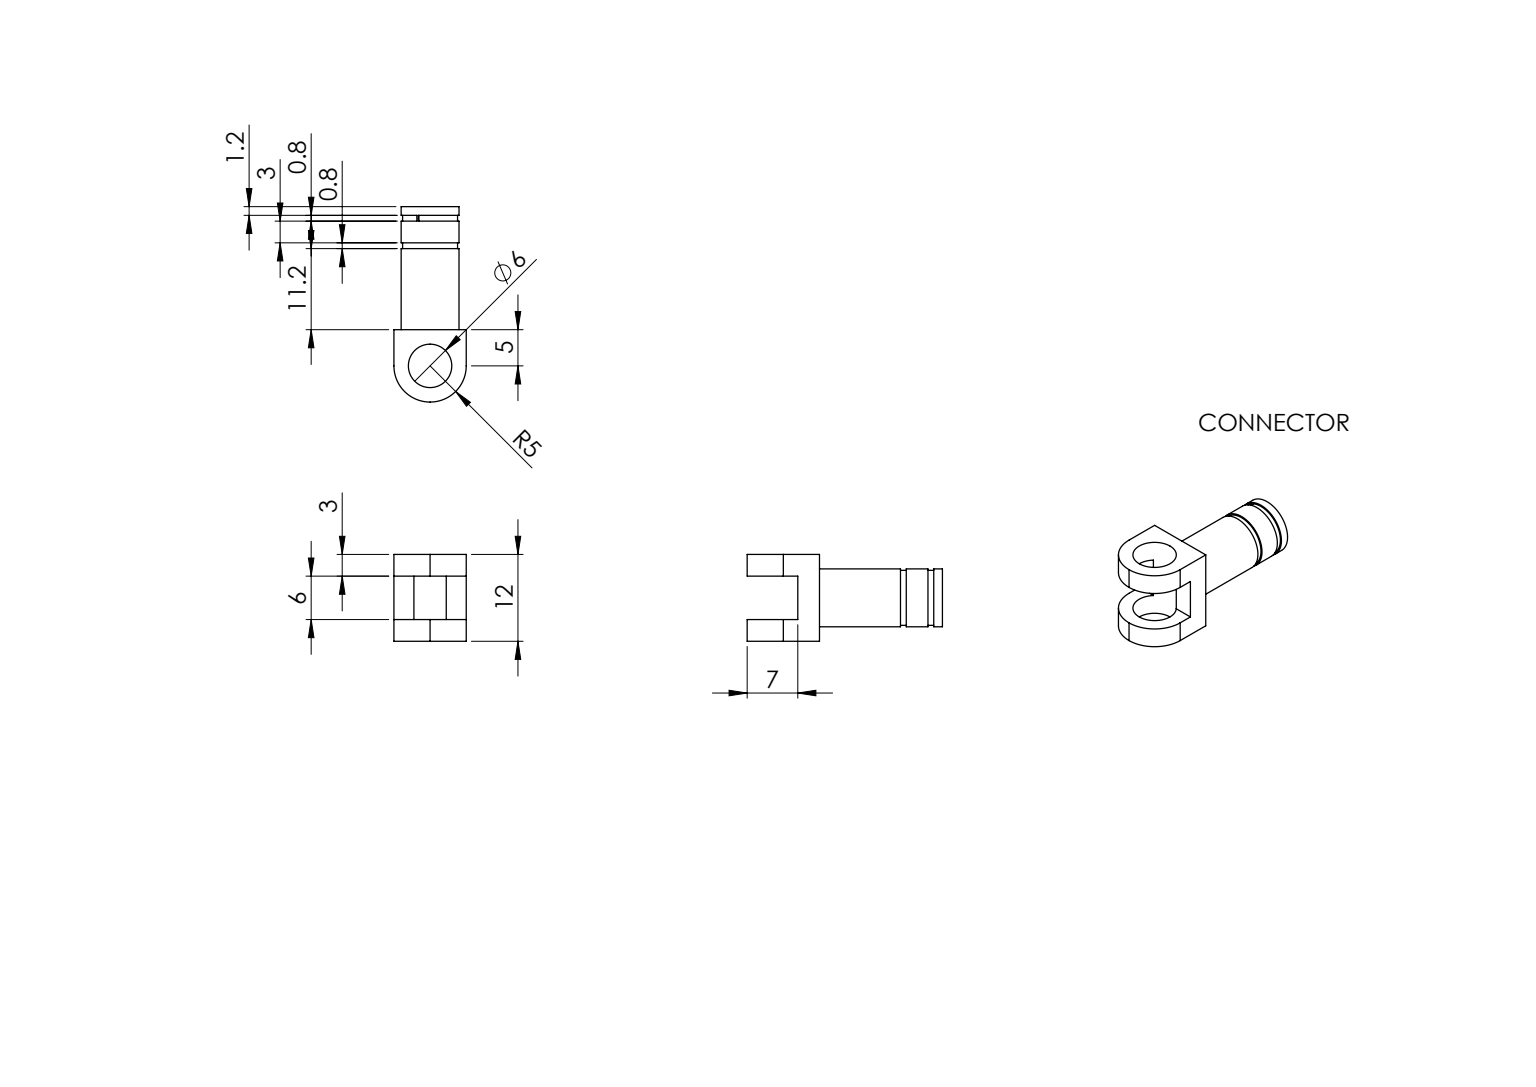
ISO-10303-21;
HEADER;
FILE_DESCRIPTION (('STEP AP214'),
    '1' );
FILE_NAME ('connector.step',
    '2026-10-31T03:41:51',
    ( '' ),
    ( '' ),
    'SwSTEP 2.0',
    'SolidWorks 2026',
    '' );
FILE_SCHEMA (( 'AUTOMOTIVE_DESIGN' ));
ENDSEC;

DATA;
#29=EDGE_CURVE ( 'NONE', #14731, #12050, #4275, .T. ) ;
#49=CARTESIAN_POINT ( 'NONE',  ( -14.40394475573011945, -10.79473832354794460, -3.794707603699265519E-15 ) ) ;
#69=ORIENTED_EDGE ( 'NONE', *, *, #13888, .F. ) ;
#80=EDGE_CURVE ( 'NONE', #14477, #12497, #893, .T. ) ;
#95=CARTESIAN_POINT ( 'NONE',  ( -14.40394475573011945, -2.082238426203170629E-15, 16.99999999999999645 ) ) ;
#102=DIRECTION ( 'NONE',  ( 0.9021244663126475327, 0.4314758942051350465, -1.141265444721583757E-16 ) ) ;
#107=VECTOR ( 'NONE', #15180, 1000.000000000000114 ) ;
#134=VERTEX_POINT ( 'NONE', #3643 ) ;
#139=CIRCLE ( 'NONE', #11189, 3.799999999999999378 ) ;
#140=EDGE_CURVE ( 'NONE', #12264, #4663, #14022, .T. ) ;
#162=CARTESIAN_POINT ( 'NONE',  ( -16.14082873121598993, -7.414910804916202913, -3.000000000000000000 ) ) ;
#189=DIRECTION ( 'NONE',  ( -1.576560579138138762E-17, 1.359337748750801608E-17, -1.000000000000000000 ) ) ;
#194=ORIENTED_EDGE ( 'NONE', *, *, #4990, .T. ) ;
#196=AXIS2_PLACEMENT_3D ( 'NONE', #5704, #8149, #10157 ) ;
#276=ORIENTED_EDGE ( 'NONE', *, *, #3938, .F. ) ;
#298=ORIENTED_EDGE ( 'NONE', *, *, #4470, .F. ) ;
#323=ORIENTED_EDGE ( 'NONE', *, *, #9187, .T. ) ;
#358=ORIENTED_EDGE ( 'NONE', *, *, #7383, .F. ) ;
#377=CARTESIAN_POINT ( 'NONE',  ( -14.40394475573011768, -13.79473832354794993, 16.99999999999999645 ) ) ;
#385=CARTESIAN_POINT ( 'NONE',  ( -16.02604379927987566, -7.138402084508245871, -3.000000000000000444 ) ) ;
#387=AXIS2_PLACEMENT_3D ( 'NONE', #8515, #438, #8738 ) ;
#415=CIRCLE ( 'NONE', #14963, 5.000000000000000888 ) ;
#416=DIRECTION ( 'NONE',  ( 1.576560579138138762E-17, -1.359337748750801608E-17, 1.000000000000000000 ) ) ;
#417=DIRECTION ( 'NONE',  ( 1.000000000000000000, 0.000000000000000000, -0.000000000000000000 ) ) ;
#418=VERTEX_POINT ( 'NONE', #1273 ) ;
#424=DIRECTION ( 'NONE',  ( -1.000000000000000000, 0.000000000000000000, -0.000000000000000000 ) ) ;
#426=CIRCLE ( 'NONE', #5853, 4.999999999999999112 ) ;
#436=DIRECTION ( 'NONE',  ( 1.000000000000000000, 0.000000000000000000, 0.000000000000000000 ) ) ;
#438=DIRECTION ( 'NONE',  ( -0.000000000000000000, -1.000000000000000000, -0.000000000000000000 ) ) ;
#453=EDGE_CURVE ( 'NONE', #2791, #11000, #13669, .T. ) ;
#490=ORIENTED_EDGE ( 'NONE', *, *, #9421, .T. ) ;
#531=CARTESIAN_POINT ( 'NONE',  ( -9.403944755730117677, -13.79473832354794816, 22.00000000000000000 ) ) ;
#532=ADVANCED_FACE ( 'NONE', ( #1053 ), #13021, .T. ) ;
#545=EDGE_CURVE ( 'NONE', #7272, #5145, #11103, .T. ) ;
#547=VECTOR ( 'NONE', #3000, 1000.000000000000000 ) ;
#598=CARTESIAN_POINT ( 'NONE',  ( -17.10144940350364706, -13.74829019802725050, -5.000000000000000000 ) ) ;
#648=DIRECTION ( 'NONE',  ( 0.000000000000000000, 0.000000000000000000, 1.000000000000000000 ) ) ;
#650=ADVANCED_FACE ( 'NONE', ( #7584 ), #3969, .T. ) ;
#653=FACE_OUTER_BOUND ( 'NONE', #7548, .T. ) ;
#667=VECTOR ( 'NONE', #8814, 999.9999999999998863 ) ;
#678=MECHANICAL_DESIGN_GEOMETRIC_PRESENTATION_REPRESENTATION('',(#1413),#6575);
#697=AXIS2_PLACEMENT_3D ( 'NONE', #7574, #6261, #2880 ) ;
#699=DIRECTION ( 'NONE',  ( 0.000000000000000000, 0.000000000000000000, 1.000000000000000000 ) ) ;
#718=DIRECTION ( 'NONE',  ( 1.445602896647338917E-16, -1.000000000000000000, 0.000000000000000000 ) ) ;
#725=ADVANCED_FACE ( 'NONE', ( #9367 ), #12746, .F. ) ;
#735=DIRECTION ( 'NONE',  ( 0.9021244663126475327, 0.4314758942051350465, -1.141265444721583757E-16 ) ) ;
#736=DIRECTION ( 'NONE',  ( -5.782411586589355667E-16, -1.000000000000000000, 0.000000000000000000 ) ) ;
#750=FACE_OUTER_BOUND ( 'NONE', #10103, .T. ) ;
#756=CARTESIAN_POINT ( 'NONE',  ( -15.94493884710238696, -7.321218896460230496, -3.800000000000000266 ) ) ;
#761=VERTEX_POINT ( 'NONE', #8286 ) ;
#782=LINE ( 'NONE', #2247, #5291 ) ;
#784=CARTESIAN_POINT ( 'NONE',  ( -14.40394475573011945, -10.79473832354794460, -3.469446951953614189E-15 ) ) ;
#819=DIRECTION ( 'NONE',  ( 1.000000000000000000, 1.445602896647338424E-16, 0.000000000000000000 ) ) ;
#830=ORIENTED_EDGE ( 'NONE', *, *, #14959, .F. ) ;
#834=ORIENTED_EDGE ( 'NONE', *, *, #13052, .F. ) ;
#851=VERTEX_POINT ( 'NONE', #7377 ) ;
#867=ORIENTED_EDGE ( 'NONE', *, *, #10936, .T. ) ;
#868=DIRECTION ( 'NONE',  ( 0.000000000000000000, 0.000000000000000000, -1.000000000000000000 ) ) ;
#880=ORIENTED_EDGE ( 'NONE', *, *, #7600, .T. ) ;
#893=CIRCLE ( 'NONE', #11692, 4.000000000000000888 ) ;
#923=CARTESIAN_POINT ( 'NONE',  ( -16.14082873121598993, -7.414910804916202913, -3.000000000000000000 ) ) ;
#928=EDGE_LOOP ( 'NONE', ( #1613, #4528 ) ) ;
#968=DIRECTION ( 'NONE',  ( 0.000000000000000000, -1.000000000000000000, 0.000000000000000000 ) ) ;
#972=EDGE_CURVE ( 'NONE', #6697, #12699, #13604, .T. ) ;
#983=ORIENTED_EDGE ( 'NONE', *, *, #14788, .T. ) ;
#988=VERTEX_POINT ( 'NONE', #5302 ) ;
#995=LINE ( 'NONE', #4236, #547 ) ;
#1006=ORIENTED_EDGE ( 'NONE', *, *, #3006, .F. ) ;
#1014=DIRECTION ( 'NONE',  ( -1.445602896647338917E-16, 1.000000000000000000, -0.000000000000000000 ) ) ;
#1022=ORIENTED_EDGE ( 'NONE', *, *, #1967, .T. ) ;
#1025=ORIENTED_EDGE ( 'NONE', *, *, #12744, .F. ) ;
#1036=LINE ( 'NONE', #6952, #3612 ) ;
#1053=FACE_OUTER_BOUND ( 'NONE', #6273, .T. ) ;
#1058=LINE ( 'NONE', #4893, #2111 ) ;
#1069=DIRECTION ( 'NONE',  ( -0.7757024858236036824, 0.6310987668242443727, 2.080818337223229247E-17 ) ) ;
#1076=FILL_AREA_STYLE ('',( #8295 ) ) ;
#1091=VECTOR ( 'NONE', #6616, 1000.000000000000000 ) ;
#1099=CARTESIAN_POINT ( 'NONE',  ( -14.40394475573011235, 8.328953704812679362E-15, 16.99999999999999645 ) ) ;
#1101=EDGE_CURVE ( 'NONE', #4663, #6635, #14169, .T. ) ;
#1107=CYLINDRICAL_SURFACE ( 'NONE', #11751, 4.000000000000000000 ) ;
#1111=DIRECTION ( 'NONE',  ( 1.576560579138138762E-17, -1.359337748750801608E-17, 1.000000000000000000 ) ) ;
#1116=AXIS2_PLACEMENT_3D ( 'NONE', #3202, #7653, #7884 ) ;
#1129=ORIENTED_EDGE ( 'NONE', *, *, #3944, .F. ) ;
#1133=FACE_BOUND ( 'NONE', #9789, .T. ) ;
#1200=CYLINDRICAL_SURFACE ( 'NONE', #10445, 5.000000000000000888 ) ;
#1219=DIRECTION ( 'NONE',  ( 0.000000000000000000, 0.000000000000000000, -1.000000000000000000 ) ) ;
#1227=CIRCLE ( 'NONE', #1977, 4.000000000000000000 ) ;
#1259=EDGE_CURVE ( 'NONE', #9849, #13077, #7974, .T. ) ;
#1270=ORIENTED_EDGE ( 'NONE', *, *, #12382, .F. ) ;
#1271=CARTESIAN_POINT ( 'NONE',  ( -14.40394475573011945, -10.79473832354794460, 0.7999999999999960476 ) ) ;
#1273=CARTESIAN_POINT ( 'NONE',  ( -9.403944755730117677, -13.79473832354794993, 16.99999999999999645 ) ) ;
#1275=VERTEX_POINT ( 'NONE', #1868 ) ;
#1285=EDGE_CURVE ( 'NONE', #14210, #12453, #13387, .T. ) ;
#1288=DIRECTION ( 'NONE',  ( 0.000000000000000000, -1.000000000000000000, 0.000000000000000000 ) ) ;
#1311=PRODUCT_DEFINITION_FORMATION_WITH_SPECIFIED_SOURCE ( 'ANY', '', #13509, .NOT_KNOWN. ) ;
#1349=DIRECTION ( 'NONE',  ( 0.000000000000000000, -1.000000000000000000, 0.000000000000000000 ) ) ;
#1359=CARTESIAN_POINT ( 'NONE',  ( -14.40394475573012301, -13.79473832354794993, 16.99999999999999645 ) ) ;
#1362=AXIS2_PLACEMENT_3D ( 'NONE', #1099, #6945, #14485 ) ;
#1376=AXIS2_PLACEMENT_3D ( 'NONE', #7353, #6187, #9640 ) ;
#1395=VECTOR ( 'NONE', #11283, 1000.000000000000000 ) ;
#1399=EDGE_CURVE ( 'NONE', #6697, #5334, #782, .T. ) ;
#1413=STYLED_ITEM('',(#15258),#13940);
#1414=ORIENTED_EDGE ( 'NONE', *, *, #6168, .F. ) ;
#1435=CARTESIAN_POINT ( 'NONE',  ( -19.40394475573011590, -4.794738323547945491, 12.00000000000000000 ) ) ;
#1441=AXIS2_PLACEMENT_3D ( 'NONE', #14034, #11793, #15127 ) ;
#1456=FACE_OUTER_BOUND ( 'NONE', #5574, .T. ) ;
#1485=VERTEX_POINT ( 'NONE', #10550 ) ;
#1490=LINE ( 'NONE', #1557, #4783 ) ;
#1491=ORIENTED_EDGE ( 'NONE', *, *, #1285, .T. ) ;
#1497=ORIENTED_EDGE ( 'NONE', *, *, #6234, .F. ) ;
#1529=LINE ( 'NONE', #7454, #4580 ) ;
#1543=EDGE_CURVE ( 'NONE', #8254, #761, #13055, .T. ) ;
#1557=CARTESIAN_POINT ( 'NONE',  ( -14.40394475573012301, -4.794738323547945491, 19.99999999999999645 ) ) ;
#1558=EDGE_CURVE ( 'NONE', #2099, #14023, #9734, .T. ) ;
#1587=AXIS2_PLACEMENT_3D ( 'NONE', #4100, #5260, #8780 ) ;
#1598=( GEOMETRIC_REPRESENTATION_CONTEXT ( 3 ) GLOBAL_UNCERTAINTY_ASSIGNED_CONTEXT ( ( #5190 ) ) GLOBAL_UNIT_ASSIGNED_CONTEXT ( ( #5513, #14057, #4970 ) ) REPRESENTATION_CONTEXT ( 'NONE', 'WORKASPACE' ) );
#1611=DIRECTION ( 'NONE',  ( -0.000000000000000000, -1.000000000000000000, -0.000000000000000000 ) ) ;
#1613=ORIENTED_EDGE ( 'NONE', *, *, #13229, .T. ) ;
#1619=CIRCLE ( 'NONE', #1856, 3.799999999999998934 ) ;
#1621=PLANE ( 'NONE',  #11146 ) ;
#1629=ORIENTED_EDGE ( 'NONE', *, *, #7674, .T. ) ;
#1644=VECTOR ( 'NONE', #11061, 1000.000000000000000 ) ;
#1664=DIRECTION ( 'NONE',  ( 0.7573544145849105957, -0.6530040510661073716, -2.081668171172162967E-17 ) ) ;
#1722=ADVANCED_FACE ( 'NONE', ( #3853 ), #11070, .F. ) ;
#1760=CARTESIAN_POINT ( 'NONE',  ( -9.403944755730117677, -16.79473832354794993, 22.00000000000000000 ) ) ;
#1809=ADVANCED_FACE ( 'NONE', ( #3165 ), #13829, .T. ) ;
#1813=VERTEX_POINT ( 'NONE', #7767 ) ;
#1817=CIRCLE ( 'NONE', #8933, 4.000000000000000000 ) ;
#1834=CARTESIAN_POINT ( 'NONE',  ( -16.64001273322991281, -7.794738323547949932, 14.99999999999999822 ) ) ;
#1846=EDGE_CURVE ( 'NONE', #3700, #6635, #6624, .T. ) ;
#1856=AXIS2_PLACEMENT_3D ( 'NONE', #6396, #6233, #3013 ) ;
#1862=CARTESIAN_POINT ( 'NONE',  ( -14.40394475573011945, -10.79473832354794460, 12.00000000000000000 ) ) ;
#1868=CARTESIAN_POINT ( 'NONE',  ( -18.40394475573011945, -10.79473832354794460, -3.406384528788088688E-15 ) ) ;
#1873=EDGE_CURVE ( 'NONE', #3107, #988, #9246, .T. ) ;
#1882=ADVANCED_FACE ( 'NONE', ( #4312 ), #10075, .F. ) ;
#1885=VERTEX_POINT ( 'NONE', #10148 ) ;
#1887=DIRECTION ( 'NONE',  ( -0.000000000000000000, -0.000000000000000000, -1.000000000000000000 ) ) ;
#1909=ORIENTED_EDGE ( 'NONE', *, *, #13404, .F. ) ;
#1926=FACE_OUTER_BOUND ( 'NONE', #4356, .T. ) ;
#1945=AXIS2_PLACEMENT_3D ( 'NONE', #10428, #416, #1664 ) ;
#1954=VECTOR ( 'NONE', #13085, 999.9999999999998863 ) ;
#1967=EDGE_CURVE ( 'NONE', #8601, #9577, #139, .T. ) ;
#1973=DIRECTION ( 'NONE',  ( 0.9021244663126475327, 0.4314758942051350465, -1.141265444721583757E-16 ) ) ;
#1975=DIRECTION ( 'NONE',  ( -5.480158469902919838E-17, -1.051478716308701618E-16, -1.000000000000000000 ) ) ;
#1977=AXIS2_PLACEMENT_3D ( 'NONE', #2826, #14447, #13201 ) ;
#1982=LINE ( 'NONE', #11413, #7043 ) ;
#2027=ORIENTED_EDGE ( 'NONE', *, *, #9884, .T. ) ;
#2040=ORIENTED_EDGE ( 'NONE', *, *, #3738, .F. ) ;
#2084=AXIS2_PLACEMENT_3D ( 'NONE', #4593, #2122, #6813 ) ;
#2092=AXIS2_PLACEMENT_3D ( 'NONE', #9331, #4571, #9393 ) ;
#2099=VERTEX_POINT ( 'NONE', #7603 ) ;
#2111=VECTOR ( 'NONE', #11579, 1000.000000000000000 ) ;
#2113=ADVANCED_FACE ( 'NONE', ( #6290 ), #14525, .F. ) ;
#2118=DIRECTION ( 'NONE',  ( 0.9021244663126475327, 0.4314758942051350465, -1.141265444721583757E-16 ) ) ;
#2122=DIRECTION ( 'NONE',  ( -1.576560579138138762E-17, 1.359337748750801608E-17, -1.000000000000000000 ) ) ;
#2152=DIRECTION ( 'NONE',  ( -5.480158469902919838E-17, -1.051478716308701618E-16, -1.000000000000000000 ) ) ;
#2167=ORIENTED_EDGE ( 'NONE', *, *, #3111, .F. ) ;
#2220=VERTEX_POINT ( 'NONE', #12514 ) ;
#2233=DIRECTION ( 'NONE',  ( 1.445602896647338917E-16, -1.000000000000000000, 0.000000000000000000 ) ) ;
#2243=CARTESIAN_POINT ( 'NONE',  ( -19.40394475573012301, -7.794738323547950820, 16.99999999999999645 ) ) ;
#2247=CARTESIAN_POINT ( 'NONE',  ( -14.40394475573011945, -4.794738323547946379, 22.00000000000000000 ) ) ;
#2252=CARTESIAN_POINT ( 'NONE',  ( -14.40394475573011945, -10.79473832354794460, -5.000000000000000000 ) ) ;
#2268=ORIENTED_EDGE ( 'NONE', *, *, #5962, .F. ) ;
#2275=DIRECTION ( 'NONE',  ( -1.445602896647338917E-16, 1.000000000000000000, -0.000000000000000000 ) ) ;
#2284=CARTESIAN_POINT ( 'NONE',  ( -14.40394475573012301, -16.79473832354794993, 16.99999999999999645 ) ) ;
#2297=EDGE_LOOP ( 'NONE', ( #4906, #13957, #12309, #12977, #13907, #1270, #11727, #7776 ) ) ;
#2302=SURFACE_SIDE_STYLE ('',( #12976 ) ) ;
#2332=DIRECTION ( 'NONE',  ( -0.000000000000000000, -1.000000000000000000, -0.000000000000000000 ) ) ;
#2333=FACE_OUTER_BOUND ( 'NONE', #13646, .T. ) ;
#2336=CYLINDRICAL_SURFACE ( 'NONE', #11386, 4.000000000000000000 ) ;
#2421=CARTESIAN_POINT ( 'NONE',  ( -10.40394475573011945, -10.79473832354794460, -3.532509375119139690E-15 ) ) ;
#2456=DIRECTION ( 'NONE',  ( -0.000000000000000000, 1.000000000000000000, -0.000000000000000000 ) ) ;
#2475=VERTEX_POINT ( 'NONE', #9728 ) ;
#2491=CARTESIAN_POINT ( 'NONE',  ( -16.23224367729419271, -7.237025146040848789, -5.000000000000000000 ) ) ;
#2543=DIRECTION ( 'NONE',  ( 0.6743761619433820131, 0.7383879686198261405, -5.947623346206184252E-19 ) ) ;
#2546=DIRECTION ( 'NONE',  ( 5.782411586589355667E-16, 1.000000000000000000, 0.000000000000000000 ) ) ;
#2558=LINE ( 'NONE', #6539, #4527 ) ;
#2571=CIRCLE ( 'NONE', #3066, 4.000000000000000000 ) ;
#2585=ORIENTED_EDGE ( 'NONE', *, *, #5962, .T. ) ;
#2608=AXIS2_PLACEMENT_3D ( 'NONE', #2988, #7751, #8897 ) ;
#2620=ADVANCED_FACE ( 'NONE', ( #14802 ), #7885, .T. ) ;
#2638=VECTOR ( 'NONE', #13736, 1000.000000000000000 ) ;
#2659=VECTOR ( 'NONE', #12856, 1000.000000000000000 ) ;
#2670=FACE_OUTER_BOUND ( 'NONE', #10290, .T. ) ;
#2676=VECTOR ( 'NONE', #1887, 1000.000000000000000 ) ;
#2684=ORIENTED_EDGE ( 'NONE', *, *, #10788, .F. ) ;
#2687=ORIENTED_EDGE ( 'NONE', *, *, #6331, .F. ) ;
#2688=CARTESIAN_POINT ( 'NONE',  ( -19.40394475573012301, -16.79473832354794993, 12.00000000000000000 ) ) ;
#2692=ORIENTED_EDGE ( 'NONE', *, *, #13890, .T. ) ;
#2703=ADVANCED_FACE ( 'NONE', ( #653 ), #12631, .T. ) ;
#2708=EDGE_CURVE ( 'NONE', #5145, #10081, #5437, .T. ) ;
#2717=PLANE ( 'NONE',  #13142 ) ;
#2719=CARTESIAN_POINT ( 'NONE',  ( -9.403944755730119454, -4.794738323547945491, 14.99999999999999822 ) ) ;
#2791=VERTEX_POINT ( 'NONE', #6950 ) ;
#2796=ORIENTED_EDGE ( 'NONE', *, *, #8740, .T. ) ;
#2797=CARTESIAN_POINT ( 'NONE',  ( -10.40394475573011945, -10.79473832354794460, 12.00000000000000000 ) ) ;
#2804=LINE ( 'NONE', #14653, #2676 ) ;
#2809=DIRECTION ( 'NONE',  ( -1.000000000000000000, -0.000000000000000000, -0.000000000000000000 ) ) ;
#2826=CARTESIAN_POINT ( 'NONE',  ( -14.40394475573011945, -10.79473832354794460, -3.469446951953614189E-15 ) ) ;
#2843=DIRECTION ( 'NONE',  ( 0.000000000000000000, -1.000000000000000000, 0.000000000000000000 ) ) ;
#2880=DIRECTION ( 'NONE',  ( 0.6743761619433820131, 0.7383879686198261405, -5.947623346206184252E-19 ) ) ;
#2881=CIRCLE ( 'NONE', #12200, 4.000000000000000000 ) ;
#2886=DIRECTION ( 'NONE',  ( 1.576560579138138762E-17, -1.359337748750801608E-17, 1.000000000000000000 ) ) ;
#2891=AXIS2_PLACEMENT_3D ( 'NONE', #12339, #14440, #424 ) ;
#2899=ORIENTED_EDGE ( 'NONE', *, *, #5713, .T. ) ;
#2902=DIRECTION ( 'NONE',  ( -0.000000000000000000, -1.000000000000000000, -0.000000000000000000 ) ) ;
#2929=EDGE_CURVE ( 'NONE', #134, #2475, #2558, .T. ) ;
#2937=EDGE_LOOP ( 'NONE', ( #11951, #5390, #3768, #9077, #3420, #14158, #8321, #10483 ) ) ;
#2947=AXIS2_PLACEMENT_3D ( 'NONE', #12814, #1288, #9302 ) ;
#2966=CARTESIAN_POINT ( 'NONE',  ( -11.52599798030746037, -13.27615371759915242, 0.7999999999999959366 ) ) ;
#2971=VERTEX_POINT ( 'NONE', #6460 ) ;
#2974=CARTESIAN_POINT ( 'NONE',  ( -16.14082873121598993, -7.414910804916202913, -3.000000000000000000 ) ) ;
#2976=SHAPE_DEFINITION_REPRESENTATION ( #5300, #10044 ) ;
#2988=CARTESIAN_POINT ( 'NONE',  ( -19.40394475573012301, -7.794738323547950820, 14.99999999999999822 ) ) ;
#2996=EDGE_CURVE ( 'NONE', #4663, #418, #6389, .T. ) ;
#3000=DIRECTION ( 'NONE',  ( 0.000000000000000000, 0.000000000000000000, -1.000000000000000000 ) ) ;
#3006=EDGE_CURVE ( 'NONE', #13883, #14059, #13088, .T. ) ;
#3013=DIRECTION ( 'NONE',  ( 0.7573544145849105957, -0.6530040510661073716, -2.853163611803960010E-17 ) ) ;
#3020=CIRCLE ( 'NONE', #10140, 3.000000000000000888 ) ;
#3035=DIRECTION ( 'NONE',  ( 0.000000000000000000, 1.000000000000000000, -1.084202172485504187E-16 ) ) ;
#3059=ORIENTED_EDGE ( 'NONE', *, *, #14913, .F. ) ;
#3066=AXIS2_PLACEMENT_3D ( 'NONE', #14467, #3933, #12294 ) ;
#3068=CARTESIAN_POINT ( 'NONE',  ( -19.40394475573012301, -7.794738323547950820, 14.99999999999999822 ) ) ;
#3077=VECTOR ( 'NONE', #6509, 999.9999999999998863 ) ;
#3106=VECTOR ( 'NONE', #10371, 1000.000000000000000 ) ;
#3107=VERTEX_POINT ( 'NONE', #923 ) ;
#3111=EDGE_CURVE ( 'NONE', #10457, #12375, #5519, .T. ) ;
#3120=DIRECTION ( 'NONE',  ( -5.480158469902919838E-17, -1.051478716308701618E-16, -1.000000000000000000 ) ) ;
#3141=DIRECTION ( 'NONE',  ( 0.000000000000000000, 0.000000000000000000, 1.000000000000000000 ) ) ;
#3156=CARTESIAN_POINT ( 'NONE',  ( -14.40394475573011945, -4.794738323547946379, 22.00000000000000000 ) ) ;
#3165=FACE_OUTER_BOUND ( 'NONE', #12101, .T. ) ;
#3167=CIRCLE ( 'NONE', #1441, 4.000000000000000888 ) ;
#3173=ORIENTED_EDGE ( 'NONE', *, *, #2929, .T. ) ;
#3195=EDGE_CURVE ( 'NONE', #12453, #8792, #5770, .T. ) ;
#3196=AXIS2_PLACEMENT_3D ( 'NONE', #13510, #7965, #11195 ) ;
#3202=CARTESIAN_POINT ( 'NONE',  ( -14.40394475573011945, -10.79473832354794460, -3.799999999999999822 ) ) ;
#3210=EDGE_LOOP ( 'NONE', ( #8081, #14742, #11925, #14374, #11488 ) ) ;
#3211=CARTESIAN_POINT ( 'NONE',  ( -18.40394475573011945, -10.79473832354794460, 12.00000000000000000 ) ) ;
#3213=CARTESIAN_POINT ( 'NONE',  ( -14.40394475573012301, -16.79473832354794993, 16.99999999999999645 ) ) ;
#3223=FACE_OUTER_BOUND ( 'NONE', #6680, .T. ) ;
#3226=ORIENTED_EDGE ( 'NONE', *, *, #11081, .T. ) ;
#3252=ADVANCED_FACE ( 'NONE', ( #6143 ), #11667, .F. ) ;
#3262=ORIENTED_EDGE ( 'NONE', *, *, #8026, .T. ) ;
#3264=CARTESIAN_POINT ( 'NONE',  ( -14.40394475573012301, -4.794738323547945491, 19.99999999999999645 ) ) ;
#3275=ADVANCED_FACE ( 'NONE', ( #1456 ), #9668, .T. ) ;
#3318=CARTESIAN_POINT ( 'NONE',  ( -14.40394475573011235, 8.328953704812679362E-15, 16.99999999999999645 ) ) ;
#3336=CARTESIAN_POINT ( 'NONE',  ( -14.40394475573011945, -10.79473832354794283, -3.000000000000000000 ) ) ;
#3372=EDGE_LOOP ( 'NONE', ( #4026, #6931, #12680, #15039 ) ) ;
#3379=CARTESIAN_POINT ( 'NONE',  ( -9.403944755730117677, -7.794738323547949044, 16.99999999999999645 ) ) ;
#3387=CARTESIAN_POINT ( 'NONE',  ( -14.40394475573012301, -7.794738323547949932, 16.99999999999999645 ) ) ;
#3417=EDGE_CURVE ( 'NONE', #9424, #14731, #8596, .T. ) ;
#3420=ORIENTED_EDGE ( 'NONE', *, *, #10811, .F. ) ;
#3437=CIRCLE ( 'NONE', #2947, 3.000000000000000888 ) ;
#3457=DIRECTION ( 'NONE',  ( -0.000000000000000000, 1.000000000000000000, -0.000000000000000000 ) ) ;
#3476=ORIENTED_EDGE ( 'NONE', *, *, #545, .F. ) ;
#3479=VERTEX_POINT ( 'NONE', #756 ) ;
#3482=DIRECTION ( 'NONE',  ( 0.000000000000000000, 0.000000000000000000, 1.000000000000000000 ) ) ;
#3489=EDGE_LOOP ( 'NONE', ( #9090, #13919, #13117, #10177, #298, #867, #4996, #9921 ) ) ;
#3496=LINE ( 'NONE', #5822, #6007 ) ;
#3514=CARTESIAN_POINT ( 'NONE',  ( -19.40394475573012301, -7.794738323547950820, 16.99999999999999645 ) ) ;
#3517=EDGE_CURVE ( 'NONE', #13077, #14623, #6897, .T. ) ;
#3520=MECHANICAL_DESIGN_GEOMETRIC_PRESENTATION_REPRESENTATION('',(#8429),#1598);
#3539=EDGE_CURVE ( 'NONE', #6635, #10618, #5457, .T. ) ;
#3563=ADVANCED_FACE ( 'NONE', ( #1133, #7196 ), #3582, .F. ) ;
#3564=CARTESIAN_POINT ( 'NONE',  ( -19.40394475573012301, -13.79473832354794993, 14.99999999999999822 ) ) ;
#3567=AXIS2_PLACEMENT_3D ( 'NONE', #9388, #11911, #2546 ) ;
#3569=CARTESIAN_POINT ( 'NONE',  ( -17.83201772771817772, -12.43434672152745613, -3.799999999999999378 ) ) ;
#3578=ORIENTED_EDGE ( 'NONE', *, *, #9884, .F. ) ;
#3582=PLANE ( 'NONE',  #14156 ) ;
#3597=ORIENTED_EDGE ( 'NONE', *, *, #7049, .F. ) ;
#3612=VECTOR ( 'NONE', #4581, 1000.000000000000000 ) ;
#3614=DIRECTION ( 'NONE',  ( 0.9021244663126474217, 0.4314758942051349910, -9.480662228539549174E-17 ) ) ;
#3626=AXIS2_PLACEMENT_3D ( 'NONE', #13734, #12507, #4279 ) ;
#3641=AXIS2_PLACEMENT_3D ( 'NONE', #11261, #6655, #735 ) ;
#3643=CARTESIAN_POINT ( 'NONE',  ( -19.40394475573012301, -13.79473832354794993, 14.99999999999999822 ) ) ;
#3654=DIRECTION ( 'NONE',  ( 0.000000000000000000, 0.000000000000000000, 1.000000000000000000 ) ) ;
#3688=DIRECTION ( 'NONE',  ( -5.480158469902917989E-17, -1.051478716308701742E-16, -1.000000000000000000 ) ) ;
#3700=VERTEX_POINT ( 'NONE', #4129 ) ;
#3710=DIRECTION ( 'NONE',  ( 1.000000000000000000, 0.000000000000000000, 0.000000000000000000 ) ) ;
#3732=ADVANCED_FACE ( 'NONE', ( #2670 ), #8493, .T. ) ;
#3735=VERTEX_POINT ( 'NONE', #2966 ) ;
#3738=EDGE_CURVE ( 'NONE', #1885, #13883, #4978, .T. ) ;
#3768=ORIENTED_EDGE ( 'NONE', *, *, #3111, .T. ) ;
#3779=ORIENTED_EDGE ( 'NONE', *, *, #4004, .T. ) ;
#3793=CARTESIAN_POINT ( 'NONE',  ( -16.23224367729419271, -7.237025146040845236, -3.000000000000000444 ) ) ;
#3829=CARTESIAN_POINT ( 'NONE',  ( -16.92833982302709828, -13.89754826684236200, -3.471826001292096363E-15 ) ) ;
#3832=DIRECTION ( 'NONE',  ( -5.480158469902919838E-17, -1.051478716308701618E-16, -1.000000000000000000 ) ) ;
#3849=AXIS2_PLACEMENT_3D ( 'NONE', #4003, #8674, #5099 ) ;
#3853=FACE_OUTER_BOUND ( 'NONE', #6301, .T. ) ;
#3866=AXIS2_PLACEMENT_3D ( 'NONE', #7153, #14378, #102 ) ;
#3904=VECTOR ( 'NONE', #15045, 1000.000000000000000 ) ;
#3918=AXIS2_PLACEMENT_3D ( 'NONE', #377, #8672, #10912 ) ;
#3933=DIRECTION ( 'NONE',  ( 1.576560579138138762E-17, -1.359337748750801608E-17, 1.000000000000000000 ) ) ;
#3938=EDGE_CURVE ( 'NONE', #14803, #9849, #1036, .T. ) ;
#3941=EDGE_LOOP ( 'NONE', ( #7656, #7213, #4630, #8940, #7923, #14872, #14071, #4635 ) ) ;
#3944=EDGE_CURVE ( 'NONE', #3945, #1275, #2881, .T. ) ;
#3945=VERTEX_POINT ( 'NONE', #2421 ) ;
#3969=CYLINDRICAL_SURFACE ( 'NONE', #12493, 3.799999999999998934 ) ;
#3973=ORIENTED_EDGE ( 'NONE', *, *, #13888, .T. ) ;
#4003=CARTESIAN_POINT ( 'NONE',  ( -16.14082873121598993, -7.414910804916202913, -3.000000000000000000 ) ) ;
#4004=EDGE_CURVE ( 'NONE', #851, #12497, #9560, .T. ) ;
#4019=EDGE_CURVE ( 'NONE', #3700, #10457, #3020, .T. ) ;
#4026=ORIENTED_EDGE ( 'NONE', *, *, #8740, .F. ) ;
#4046=DIRECTION ( 'NONE',  ( 0.000000000000000000, 0.000000000000000000, 1.000000000000000000 ) ) ;
#4049=CIRCLE ( 'NONE', #7971, 3.000000000000000888 ) ;
#4054=CYLINDRICAL_SURFACE ( 'NONE', #6084, 3.000000000000000888 ) ;
#4067=EDGE_LOOP ( 'NONE', ( #13062, #11992, #7774, #1629 ) ) ;
#4073=VECTOR ( 'NONE', #7837, 1000.000000000000000 ) ;
#4078=DIRECTION ( 'NONE',  ( -1.576560579138138762E-17, 1.359337748750801608E-17, -1.000000000000000000 ) ) ;
#4094=UNCERTAINTY_MEASURE_WITH_UNIT (LENGTH_MEASURE( 1.000000000000000082E-05 ), #10539, 'distance_accuracy_value', 'NONE');
#4100=CARTESIAN_POINT ( 'NONE',  ( -14.40394475573011945, -10.79473832354794460, -3.794707603699265519E-15 ) ) ;
#4129=CARTESIAN_POINT ( 'NONE',  ( -12.16787677823033142, -7.794738323547949932, 14.99999999999999822 ) ) ;
#4142=DIRECTION ( 'NONE',  ( 1.000000000000000000, 0.000000000000000000, 0.000000000000000000 ) ) ;
#4144=DIRECTION ( 'NONE',  ( 1.576560579138138762E-17, -1.359337748750801608E-17, 1.000000000000000000 ) ) ;
#4184=DIRECTION ( 'NONE',  ( 1.576560579138138762E-17, -1.359337748750801608E-17, 1.000000000000000000 ) ) ;
#4200=DIRECTION ( 'NONE',  ( -0.000000000000000000, -1.000000000000000000, -0.000000000000000000 ) ) ;
#4201=DIRECTION ( 'NONE',  ( 0.000000000000000000, 0.000000000000000000, 1.000000000000000000 ) ) ;
#4210=LINE ( 'NONE', #7736, #4612 ) ;
#4217=EDGE_CURVE ( 'NONE', #5125, #134, #5351, .T. ) ;
#4236=CARTESIAN_POINT ( 'NONE',  ( -19.40394475573012301, -13.79473832354794993, 16.99999999999999645 ) ) ;
#4238=CARTESIAN_POINT ( 'NONE',  ( -15.94493884710238696, -7.321218896460230496, -3.000000000000000000 ) ) ;
#4255=DIRECTION ( 'NONE',  ( 1.000000000000000000, 1.734723475976807341E-16, 2.081668171172168908E-15 ) ) ;
#4275=LINE ( 'NONE', #14736, #10383 ) ;
#4279=DIRECTION ( 'NONE',  ( 0.000000000000000000, 1.000000000000000000, -1.084202172485504187E-16 ) ) ;
#4312=FACE_OUTER_BOUND ( 'NONE', #12524, .T. ) ;
#4338=CARTESIAN_POINT ( 'NONE',  ( -10.97587178374205941, -9.155129925568431304, -3.000000000000000444 ) ) ;
#4356=EDGE_LOOP ( 'NONE', ( #14181, #9341, #11503, #9338, #8459 ) ) ;
#4394=DIRECTION ( 'NONE',  ( 0.9021244663126474217, 0.4314758942051349910, -9.480662228539549174E-17 ) ) ;
#4408=VECTOR ( 'NONE', #2809, 1000.000000000000000 ) ;
#4409=VECTOR ( 'NONE', #11012, 1000.000000000000000 ) ;
#4470=EDGE_CURVE ( 'NONE', #10878, #134, #995, .T. ) ;
#4479=LINE ( 'NONE', #9160, #6865 ) ;
#4498=CYLINDRICAL_SURFACE ( 'NONE', #9794, 3.799999999999999378 ) ;
#4514=CARTESIAN_POINT ( 'NONE',  ( -19.40394475573011590, -4.794738323547945491, 16.99999999999999645 ) ) ;
#4523=CARTESIAN_POINT ( 'NONE',  ( -12.16787677823033142, -13.79473832354794993, 14.99999999999999822 ) ) ;
#4524=CARTESIAN_POINT ( 'NONE',  ( -16.92833982302709828, -13.89754826684236200, 0.7999999999999960476 ) ) ;
#4527=VECTOR ( 'NONE', #11071, 1000.000000000000000 ) ;
#4528=ORIENTED_EDGE ( 'NONE', *, *, #12744, .T. ) ;
#4550=CARTESIAN_POINT ( 'NONE',  ( -14.40394475573011945, -10.79473832354794460, -5.000000000000000000 ) ) ;
#4551=CIRCLE ( 'NONE', #2084, 3.799999999999998934 ) ;
#4557=DIRECTION ( 'NONE',  ( -5.480158469902919838E-17, -1.051478716308701618E-16, -1.000000000000000000 ) ) ;
#4571=DIRECTION ( 'NONE',  ( 1.576560579138138762E-17, -1.359337748750801762E-17, 1.000000000000000000 ) ) ;
#4580=VECTOR ( 'NONE', #1611, 1000.000000000000000 ) ;
#4581=DIRECTION ( 'NONE',  ( 0.6743761619433820131, 0.7383879686198261405, -5.947623346206184252E-19 ) ) ;
#4584=EDGE_LOOP ( 'NONE', ( #9033, #11682, #11208, #14116, #11428, #13711, #10453, #2167 ) ) ;
#4593=CARTESIAN_POINT ( 'NONE',  ( -14.40394475573011945, -10.79473832354794460, 0.7999999999999960476 ) ) ;
#4612=VECTOR ( 'NONE', #13648, 1000.000000000000000 ) ;
#4630=ORIENTED_EDGE ( 'NONE', *, *, #13966, .T. ) ;
#4635=ORIENTED_EDGE ( 'NONE', *, *, #4019, .T. ) ;
#4650=CARTESIAN_POINT ( 'NONE',  ( -10.40394475573011945, -10.79473832354794460, 0.7999999999999959366 ) ) ;
#4655=PLANE ( 'NONE',  #2092 ) ;
#4663=VERTEX_POINT ( 'NONE', #10889 ) ;
#4757=LINE ( 'NONE', #4920, #9449 ) ;
#4781=CARTESIAN_POINT ( 'NONE',  ( -14.40394475573011945, -10.79473832354794283, -3.799999999999999822 ) ) ;
#4783=VECTOR ( 'NONE', #7484, 1000.000000000000000 ) ;
#4815=CARTESIAN_POINT ( 'NONE',  ( -17.83201772771817772, -12.43434672152745613, -2.999999999999999556 ) ) ;
#4822=EDGE_LOOP ( 'NONE', ( #11425, #3597, #7785, #3476 ) ) ;
#4825=DIRECTION ( 'NONE',  ( 0.000000000000000000, 0.000000000000000000, -1.000000000000000000 ) ) ;
#4836=DIRECTION ( 'NONE',  ( 0.000000000000000000, 1.000000000000000000, 0.000000000000000000 ) ) ;
#4893=CARTESIAN_POINT ( 'NONE',  ( -9.403944755730119454, -4.794738323547945491, 22.00000000000000000 ) ) ;
#4902=AXIS2_PLACEMENT_3D ( 'NONE', #10449, #1069, #14051 ) ;
#4906=ORIENTED_EDGE ( 'NONE', *, *, #1101, .F. ) ;
#4912=ADVANCED_BREP_SHAPE_REPRESENTATION ( '', ( #13940, #1376 ), #9175 ) ;
#4913=CIRCLE ( 'NONE', #3918, 4.999999999999999112 ) ;
#4920=CARTESIAN_POINT ( 'NONE',  ( -12.16787677823033142, -4.794738323547945491, 14.99999999999999822 ) ) ;
#4927=LINE ( 'NONE', #9596, #14190 ) ;
#4932=PRESENTATION_STYLE_ASSIGNMENT (( #5988 ) ) ;
#4944=ORIENTED_EDGE ( 'NONE', *, *, #10881, .F. ) ;
#4949=ORIENTED_EDGE ( 'NONE', *, *, #1846, .F. ) ;
#4955=VECTOR ( 'NONE', #718, 1000.000000000000000 ) ;
#4970=( NAMED_UNIT ( * ) SI_UNIT ( $, .STERADIAN. ) SOLID_ANGLE_UNIT ( ) );
#4971=DIRECTION ( 'NONE',  ( 1.445602896647338917E-16, -1.000000000000000000, 0.000000000000000000 ) ) ;
#4978=LINE ( 'NONE', #9648, #9257 ) ;
#4990=EDGE_CURVE ( 'NONE', #9577, #3479, #5897, .T. ) ;
#4996=ORIENTED_EDGE ( 'NONE', *, *, #5458, .T. ) ;
#5016=VERTEX_POINT ( 'NONE', #9347 ) ;
#5018=CARTESIAN_POINT ( 'NONE',  ( -16.96657417111497068, -13.60061260430328467, 0.7999999999999960476 ) ) ;
#5060=EDGE_CURVE ( 'NONE', #851, #2099, #7356, .T. ) ;
#5066=DIRECTION ( 'NONE',  ( 0.000000000000000000, 0.000000000000000000, 1.000000000000000000 ) ) ;
#5080=CARTESIAN_POINT ( 'NONE',  ( -16.80212006966224791, -13.74240776967763900, -3.794707603699265519E-15 ) ) ;
#5081=EDGE_CURVE ( 'NONE', #12694, #14059, #12022, .T. ) ;
#5084=APPLICATION_CONTEXT ( 'automotive_design' ) ;
#5089=ORIENTED_EDGE ( 'NONE', *, *, #9187, .F. ) ;
#5090=DIRECTION ( 'NONE',  ( 1.000000000000000000, 0.000000000000000000, 0.000000000000000000 ) ) ;
#5095=VECTOR ( 'NONE', #9131, 1000.000000000000000 ) ;
#5099=DIRECTION ( 'NONE',  ( 0.4570747303910189796, -0.8894282943767739535, 6.847307257068339928E-17 ) ) ;
#5100=CIRCLE ( 'NONE', #5586, 4.000000000000000000 ) ;
#5106=ORIENTED_EDGE ( 'NONE', *, *, #10673, .T. ) ;
#5125=VERTEX_POINT ( 'NONE', #6469 ) ;
#5145=VERTEX_POINT ( 'NONE', #10802 ) ;
#5174=CARTESIAN_POINT ( 'NONE',  ( -18.40394475573011945, -10.79473832354794460, -2.999999999999999556 ) ) ;
#5175=CARTESIAN_POINT ( 'NONE',  ( -14.40394475573012301, -7.794738323547949932, 20.00000000000000000 ) ) ;
#5190=UNCERTAINTY_MEASURE_WITH_UNIT (LENGTH_MEASURE( 1.000000000000000082E-05 ), #5513, 'distance_accuracy_value', 'NONE');
#5248=ADVANCED_FACE ( 'NONE', ( #6701 ), #14856, .T. ) ;
#5260=DIRECTION ( 'NONE',  ( -1.576560579138138762E-17, 1.359337748750801608E-17, -1.000000000000000000 ) ) ;
#5291=VECTOR ( 'NONE', #1014, 1000.000000000000000 ) ;
#5294=FACE_OUTER_BOUND ( 'NONE', #4067, .T. ) ;
#5300=PRODUCT_DEFINITION_SHAPE ( 'NONE', 'NONE',  #6837 ) ;
#5302=CARTESIAN_POINT ( 'NONE',  ( -17.83201772771817772, -12.43434672152745613, -2.999999999999999556 ) ) ;
#5318=AXIS2_PLACEMENT_3D ( 'NONE', #2252, #868, #14865 ) ;
#5323=EDGE_CURVE ( 'NONE', #8601, #1485, #4479, .T. ) ;
#5327=CARTESIAN_POINT ( 'NONE',  ( -14.40394475573011945, -10.79473832354794460, 12.00000000000000000 ) ) ;
#5334=VERTEX_POINT ( 'NONE', #6632 ) ;
#5338=VECTOR ( 'NONE', #11247, 1000.000000000000000 ) ;
#5351=LINE ( 'NONE', #13707, #4955 ) ;
#5372=VECTOR ( 'NONE', #436, 1000.000000000000000 ) ;
#5376=ORIENTED_EDGE ( 'NONE', *, *, #8164, .T. ) ;
#5383=FACE_OUTER_BOUND ( 'NONE', #3210, .T. ) ;
#5390=ORIENTED_EDGE ( 'NONE', *, *, #7607, .T. ) ;
#5392=AXIS2_PLACEMENT_3D ( 'NONE', #1271, #189, #13968 ) ;
#5414=DIRECTION ( 'NONE',  ( 0.000000000000000000, 0.000000000000000000, -1.000000000000000000 ) ) ;
#5437=LINE ( 'NONE', #14656, #8386 ) ;
#5451=PLANE ( 'NONE',  #13253 ) ;
#5457=LINE ( 'NONE', #15051, #5095 ) ;
#5458=EDGE_CURVE ( 'NONE', #5334, #418, #4913, .T. ) ;
#5461=CARTESIAN_POINT ( 'NONE',  ( -14.40394475573012301, -13.79473832354794993, 20.00000000000000000 ) ) ;
#5493=DIRECTION ( 'NONE',  ( 1.000000000000000000, 0.000000000000000000, -1.576560579138137530E-17 ) ) ;
#5513=( LENGTH_UNIT ( ) NAMED_UNIT ( * ) SI_UNIT ( .MILLI., .METRE. ) );
#5519=CIRCLE ( 'NONE', #6479, 3.000000000000000888 ) ;
#5531=ORIENTED_EDGE ( 'NONE', *, *, #6724, .T. ) ;
#5558=EDGE_LOOP ( 'NONE', ( #9446, #11851, #490, #7750 ) ) ;
#5574=EDGE_LOOP ( 'NONE', ( #7452, #11220, #2692, #13629 ) ) ;
#5586=AXIS2_PLACEMENT_3D ( 'NONE', #4550, #9231, #13920 ) ;
#5593=CARTESIAN_POINT ( 'NONE',  ( -14.40394475573011768, -7.794738323547949932, 16.99999999999999645 ) ) ;
#5598=DIRECTION ( 'NONE',  ( 1.576560579138138762E-17, -1.359337748750801608E-17, 1.000000000000000000 ) ) ;
#5603=DIRECTION ( 'NONE',  ( 0.7573544145849104847, -0.6530040510661075936, -2.081668171172168513E-17 ) ) ;
#5669=DIRECTION ( 'NONE',  ( 0.000000000000000000, 0.000000000000000000, -1.000000000000000000 ) ) ;
#5695=DIRECTION ( 'NONE',  ( -5.480158469902917989E-17, -1.051478716308701742E-16, -1.000000000000000000 ) ) ;
#5699=EDGE_CURVE ( 'NONE', #15019, #14477, #8324, .T. ) ;
#5704=CARTESIAN_POINT ( 'NONE',  ( -14.40394475573012301, -4.794738323547945491, 16.99999999999999645 ) ) ;
#5713=EDGE_CURVE ( 'NONE', #12819, #13750, #3437, .T. ) ;
#5770=CIRCLE ( 'NONE', #6989, 5.000000000000000888 ) ;
#5799=FACE_OUTER_BOUND ( 'NONE', #10338, .T. ) ;
#5802=CARTESIAN_POINT ( 'NONE',  ( -14.40394475573012301, -16.79473832354794993, 16.99999999999999645 ) ) ;
#5811=DIRECTION ( 'NONE',  ( 1.000000000000000000, 1.445602896647338917E-16, -0.000000000000000000 ) ) ;
#5817=EDGE_CURVE ( 'NONE', #8792, #9979, #7617, .T. ) ;
#5820=VECTOR ( 'NONE', #2543, 1000.000000000000000 ) ;
#5822=CARTESIAN_POINT ( 'NONE',  ( -9.403944755730119454, -4.794738323547945491, 12.00000000000000000 ) ) ;
#5827=VECTOR ( 'NONE', #5811, 1000.000000000000000 ) ;
#5853=AXIS2_PLACEMENT_3D ( 'NONE', #13066, #12544, #4255 ) ;
#5864=EDGE_CURVE ( 'NONE', #8779, #2220, #11963, .T. ) ;
#5883=CARTESIAN_POINT ( 'NONE',  ( -14.40394475573011945, -10.79473832354794460, -5.000000000000000000 ) ) ;
#5887=CARTESIAN_POINT ( 'NONE',  ( -14.40394475573011945, -10.79473832354794460, -3.469446951953614189E-15 ) ) ;
#5897=LINE ( 'NONE', #14106, #3904 ) ;
#5923=CARTESIAN_POINT ( 'NONE',  ( -19.40394475573012301, -13.79473832354794993, 16.99999999999999645 ) ) ;
#5957=CARTESIAN_POINT ( 'NONE',  ( -19.40394475573012301, -16.79473832354794993, 12.00000000000000000 ) ) ;
#5962=EDGE_CURVE ( 'NONE', #7105, #3945, #1227, .T. ) ;
#5967=DIRECTION ( 'NONE',  ( -0.000000000000000000, 0.000000000000000000, 1.000000000000000000 ) ) ;
#5974=CARTESIAN_POINT ( 'NONE',  ( -17.10144940350364706, -13.74829019802725050, -3.467067902615131620E-15 ) ) ;
#5988=SURFACE_STYLE_USAGE ( .BOTH. , #2302 ) ;
#6006=ADVANCED_FACE ( 'NONE', ( #6599, #5383 ), #6512, .F. ) ;
#6007=VECTOR ( 'NONE', #2275, 1000.000000000000000 ) ;
#6021=ADVANCED_FACE ( 'NONE', ( #750 ), #5451, .F. ) ;
#6025=DIRECTION ( 'NONE',  ( 0.000000000000000000, 0.000000000000000000, 1.000000000000000000 ) ) ;
#6039=CARTESIAN_POINT ( 'NONE',  ( -14.40394475573011945, -10.79473832354794460, 0.7999999999999960476 ) ) ;
#6079=ADVANCED_FACE ( 'NONE', ( #13739 ), #6739, .T. ) ;
#6084=AXIS2_PLACEMENT_3D ( 'NONE', #13421, #2902, #12270 ) ;
#6085=DIRECTION ( 'NONE',  ( 0.9021244663126475327, 0.4314758942051350465, -1.141265444721583757E-16 ) ) ;
#6097=CYLINDRICAL_SURFACE ( 'NONE', #1362, 5.000000000000000888 ) ;
#6115=PLANE ( 'NONE',  #697 ) ;
#6127=AXIS2_PLACEMENT_3D ( 'NONE', #7763, #2152, #6840 ) ;
#6131=CARTESIAN_POINT ( 'NONE',  ( -15.94493884710238696, -7.321218896460230496, -3.000000000000000000 ) ) ;
#6143=FACE_OUTER_BOUND ( 'NONE', #3489, .T. ) ;
#6168=EDGE_CURVE ( 'NONE', #12699, #10878, #15046, .T. ) ;
#6187=DIRECTION ( 'NONE',  ( 0.000000000000000000, 0.000000000000000000, 1.000000000000000000 ) ) ;
#6226=PLANE ( 'NONE',  #7720 ) ;
#6233=DIRECTION ( 'NONE',  ( -1.576560579138138762E-17, 1.359337748750801608E-17, -1.000000000000000000 ) ) ;
#6234=EDGE_CURVE ( 'NONE', #12050, #12694, #14180, .T. ) ;
#6241=DIRECTION ( 'NONE',  ( -1.000000000000000000, -1.445602896647338917E-16, 0.000000000000000000 ) ) ;
#6251=ORIENTED_EDGE ( 'NONE', *, *, #14650, .F. ) ;
#6255=CARTESIAN_POINT ( 'NONE',  ( -11.52599798030746037, -13.27615371759915242, -3.873810994203807765E-15 ) ) ;
#6260=AXIS2_PLACEMENT_3D ( 'NONE', #10275, #5598, #11274 ) ;
#6261=DIRECTION ( 'NONE',  ( 0.7383879686198261405, -0.6743761619433820131, -2.080818337223229863E-17 ) ) ;
#6273=EDGE_LOOP ( 'NONE', ( #12955, #12182, #10329, #10999 ) ) ;
#6290=FACE_OUTER_BOUND ( 'NONE', #2937, .T. ) ;
#6300=ORIENTED_EDGE ( 'NONE', *, *, #8164, .F. ) ;
#6301=EDGE_LOOP ( 'NONE', ( #11970, #7537, #3059, #9167 ) ) ;
#6302=LINE ( 'NONE', #598, #1644 ) ;
#6315=ORIENTED_EDGE ( 'NONE', *, *, #1259, .T. ) ;
#6327=CARTESIAN_POINT ( 'NONE',  ( -9.403944755730117677, -7.794738323547949044, 14.99999999999999822 ) ) ;
#6331=EDGE_CURVE ( 'NONE', #12699, #10081, #2804, .T. ) ;
#6338=VERTEX_POINT ( 'NONE', #6576 ) ;
#6384=EDGE_CURVE ( 'NONE', #2971, #6697, #415, .T. ) ;
#6389=LINE ( 'NONE', #531, #11627 ) ;
#6391=EDGE_CURVE ( 'NONE', #2220, #1813, #14472, .T. ) ;
#6394=ORIENTED_EDGE ( 'NONE', *, *, #3006, .T. ) ;
#6396=CARTESIAN_POINT ( 'NONE',  ( -14.40394475573011945, -10.79473832354794460, 0.7999999999999960476 ) ) ;
#6446=ORIENTED_EDGE ( 'NONE', *, *, #4470, .T. ) ;
#6454=FACE_OUTER_BOUND ( 'NONE', #4584, .T. ) ;
#6460=CARTESIAN_POINT ( 'NONE',  ( -9.403944755730117677, -16.79473832354794993, 16.99999999999999645 ) ) ;
#6469=CARTESIAN_POINT ( 'NONE',  ( -19.40394475573012301, -7.794738323547950820, 14.99999999999999822 ) ) ;
#6479=AXIS2_PLACEMENT_3D ( 'NONE', #3387, #2233, #11445 ) ;
#6492=CARTESIAN_POINT ( 'NONE',  ( -14.40394475573011768, -16.79473832354794993, 16.99999999999999645 ) ) ;
#6509=DIRECTION ( 'NONE',  ( -0.4055247608874392173, 0.9140840597599245720, -7.389059384413459453E-17 ) ) ;
#6512=PLANE ( 'NONE',  #3196 ) ;
#6539=CARTESIAN_POINT ( 'NONE',  ( -19.40394475573012301, -13.79473832354794993, 14.99999999999999822 ) ) ;
#6564=VECTOR ( 'NONE', #8201, 999.9999999999998863 ) ;
#6572=ADVANCED_FACE ( 'NONE', ( #11556 ), #4498, .T. ) ;
#6575=( GEOMETRIC_REPRESENTATION_CONTEXT ( 3 ) GLOBAL_UNCERTAINTY_ASSIGNED_CONTEXT ( ( #9237 ) ) GLOBAL_UNIT_ASSIGNED_CONTEXT ( ( #12640, #6809, #12505 ) ) REPRESENTATION_CONTEXT ( 'NONE', 'WORKASPACE' ) );
#6576=CARTESIAN_POINT ( 'NONE',  ( -10.40394475573011945, -10.79473832354794460, -5.000000000000000000 ) ) ;
#6591=DIRECTION ( 'NONE',  ( 5.480158469902919838E-17, 1.051478716308701618E-16, 1.000000000000000000 ) ) ;
#6599=FACE_BOUND ( 'NONE', #9133, .T. ) ;
#6612=ADVANCED_FACE ( 'NONE', ( #2333 ), #1107, .T. ) ;
#6616=DIRECTION ( 'NONE',  ( -0.000000000000000000, -0.000000000000000000, -1.000000000000000000 ) ) ;
#6624=LINE ( 'NONE', #13762, #3106 ) ;
#6632=CARTESIAN_POINT ( 'NONE',  ( -14.40394475573011945, -13.79473832354794993, 22.00000000000000000 ) ) ;
#6634=EDGE_CURVE ( 'NONE', #3107, #2099, #13156, .T. ) ;
#6635=VERTEX_POINT ( 'NONE', #6327 ) ;
#6655=DIRECTION ( 'NONE',  ( 5.480158469902919838E-17, 1.051478716308701618E-16, 1.000000000000000000 ) ) ;
#6659=DIRECTION ( 'NONE',  ( 0.000000000000000000, 1.000000000000000000, -1.084202172485504187E-16 ) ) ;
#6666=CARTESIAN_POINT ( 'NONE',  ( -10.40394475573011945, -10.79473832354794460, -3.000000000000000444 ) ) ;
#6670=CARTESIAN_POINT ( 'NONE',  ( -14.40394475573011945, -10.79473832354794460, 0.7999999999999960476 ) ) ;
#6680=EDGE_LOOP ( 'NONE', ( #13494, #14460, #7445, #3173 ) ) ;
#6697=VERTEX_POINT ( 'NONE', #12999 ) ;
#6701=FACE_OUTER_BOUND ( 'NONE', #5558, .T. ) ;
#6722=ORIENTED_EDGE ( 'NONE', *, *, #3738, .T. ) ;
#6724=EDGE_CURVE ( 'NONE', #5016, #10618, #426, .T. ) ;
#6735=AXIS2_PLACEMENT_3D ( 'NONE', #5327, #8840, #7691 ) ;
#6739=CYLINDRICAL_SURFACE ( 'NONE', #8102, 3.799999999999998934 ) ;
#6742=DIRECTION ( 'NONE',  ( 1.445602896647338917E-16, -1.000000000000000000, 0.000000000000000000 ) ) ;
#6772=ORIENTED_EDGE ( 'NONE', *, *, #4990, .F. ) ;
#6808=ORIENTED_EDGE ( 'NONE', *, *, #140, .T. ) ;
#6809=( NAMED_UNIT ( * ) PLANE_ANGLE_UNIT ( ) SI_UNIT ( $, .RADIAN. ) );
#6811=CIRCLE ( 'NONE', #8773, 4.999999999999999112 ) ;
#6813=DIRECTION ( 'NONE',  ( 0.7573544145849105957, -0.6530040510661073716, -2.853163611803960010E-17 ) ) ;
#6837=PRODUCT_DEFINITION ( 'UNKNOWN', '', #1311, #8687 ) ;
#6840=DIRECTION ( 'NONE',  ( 0.000000000000000000, 1.000000000000000000, -1.084202172485504187E-16 ) ) ;
#6865=VECTOR ( 'NONE', #4557, 1000.000000000000000 ) ;
#6869=LINE ( 'NONE', #10477, #107 ) ;
#6893=ORIENTED_EDGE ( 'NONE', *, *, #10084, .F. ) ;
#6897=LINE ( 'NONE', #11575, #1395 ) ;
#6902=ORIENTED_EDGE ( 'NONE', *, *, #8026, .F. ) ;
#6917=DIRECTION ( 'NONE',  ( 5.480158469902919838E-17, 1.051478716308701618E-16, 1.000000000000000000 ) ) ;
#6931=ORIENTED_EDGE ( 'NONE', *, *, #3417, .T. ) ;
#6945=DIRECTION ( 'NONE',  ( 5.782411586589355667E-16, 1.000000000000000000, 0.000000000000000000 ) ) ;
#6950=CARTESIAN_POINT ( 'NONE',  ( -14.40394475573012301, -16.79473832354794993, 13.99999999999999645 ) ) ;
#6952=CARTESIAN_POINT ( 'NONE',  ( -16.96657417111497068, -13.60061260430328467, -3.794707603699265519E-15 ) ) ;
#6979=CARTESIAN_POINT ( 'NONE',  ( -9.403944755730117677, -16.79473832354794993, 16.99999999999999645 ) ) ;
#6989=AXIS2_PLACEMENT_3D ( 'NONE', #13991, #3457, #11302 ) ;
#6993=EDGE_LOOP ( 'NONE', ( #8617, #6446, #10269, #12887, #1491, #12622, #8690, #2687 ) ) ;
#6994=ORIENTED_EDGE ( 'NONE', *, *, #6391, .T. ) ;
#6997=CIRCLE ( 'NONE', #10429, 4.999999999999999112 ) ;
#7007=EDGE_CURVE ( 'NONE', #9849, #761, #4927, .T. ) ;
#7020=DIRECTION ( 'NONE',  ( 1.000000000000000000, 0.000000000000000000, 0.000000000000000000 ) ) ;
#7043=VECTOR ( 'NONE', #13877, 1000.000000000000000 ) ;
#7049=EDGE_CURVE ( 'NONE', #10081, #9211, #12115, .T. ) ;
#7058=CIRCLE ( 'NONE', #196, 3.000000000000000888 ) ;
#7059=AXIS2_PLACEMENT_3D ( 'NONE', #14873, #3120, #3035 ) ;
#7086=AXIS2_PLACEMENT_3D ( 'NONE', #2284, #1349, #4825 ) ;
#7105=VERTEX_POINT ( 'NONE', #3829 ) ;
#7140=DIRECTION ( 'NONE',  ( 0.000000000000000000, 0.000000000000000000, -1.000000000000000000 ) ) ;
#7153=CARTESIAN_POINT ( 'NONE',  ( -14.40394475573011945, -10.79473832354794283, -3.799999999999999822 ) ) ;
#7169=ORIENTED_EDGE ( 'NONE', *, *, #9165, .F. ) ;
#7174=CARTESIAN_POINT ( 'NONE',  ( -18.40394475573011945, -10.79473832354794460, -3.799999999999999378 ) ) ;
#7196=FACE_OUTER_BOUND ( 'NONE', #4822, .T. ) ;
#7213=ORIENTED_EDGE ( 'NONE', *, *, #9029, .F. ) ;
#7215=DIRECTION ( 'NONE',  ( 5.480158469902919838E-17, 1.051478716308701618E-16, 1.000000000000000000 ) ) ;
#7222=ORIENTED_EDGE ( 'NONE', *, *, #3938, .T. ) ;
#7228=ADVANCED_FACE ( 'NONE', ( #11349 ), #11198, .T. ) ;
#7235=DIRECTION ( 'NONE',  ( 5.480158469902919838E-17, 1.051478716308701618E-16, 1.000000000000000000 ) ) ;
#7272=VERTEX_POINT ( 'NONE', #12648 ) ;
#7294=DIRECTION ( 'NONE',  ( 1.576560579138138762E-17, -1.359337748750801608E-17, 1.000000000000000000 ) ) ;
#7298=DIRECTION ( 'NONE',  ( 1.000000000000000000, 1.445602896647338917E-16, 0.000000000000000000 ) ) ;
#7322=EDGE_CURVE ( 'NONE', #7692, #851, #3167, .T. ) ;
#7353=CARTESIAN_POINT ( 'NONE',  ( 0.000000000000000000, 0.000000000000000000, 0.000000000000000000 ) ) ;
#7356=LINE ( 'NONE', #10727, #1954 ) ;
#7368=CARTESIAN_POINT ( 'NONE',  ( -14.40394475573011945, -10.79473832354794460, -5.000000000000000000 ) ) ;
#7377=CARTESIAN_POINT ( 'NONE',  ( -16.23224367729419271, -7.237025146040845236, -3.800000000000000266 ) ) ;
#7378=AXIS2_PLACEMENT_3D ( 'NONE', #12967, #2456, #7140 ) ;
#7383=EDGE_CURVE ( 'NONE', #14623, #3735, #11985, .T. ) ;
#7401=EDGE_LOOP ( 'NONE', ( #11031, #1414, #9162, #12268 ) ) ;
#7406=CARTESIAN_POINT ( 'NONE',  ( -9.403944755730119454, -4.794738323547945491, 22.00000000000000000 ) ) ;
#7444=VECTOR ( 'NONE', #6025, 1000.000000000000000 ) ;
#7445=ORIENTED_EDGE ( 'NONE', *, *, #4217, .T. ) ;
#7452=ORIENTED_EDGE ( 'NONE', *, *, #7600, .F. ) ;
#7454=CARTESIAN_POINT ( 'NONE',  ( -16.64001273322991281, -4.794738323547945491, 14.99999999999999822 ) ) ;
#7484=DIRECTION ( 'NONE',  ( -0.000000000000000000, -1.000000000000000000, -0.000000000000000000 ) ) ;
#7530=AXIS2_PLACEMENT_3D ( 'NONE', #14771, #5695, #4394 ) ;
#7537=ORIENTED_EDGE ( 'NONE', *, *, #6634, .F. ) ;
#7544=AXIS2_PLACEMENT_3D ( 'NONE', #13141, #7235, #6085 ) ;
#7548=EDGE_LOOP ( 'NONE', ( #6893, #11644, #10604, #7925 ) ) ;
#7560=ORIENTED_EDGE ( 'NONE', *, *, #11140, .T. ) ;
#7574=CARTESIAN_POINT ( 'NONE',  ( -16.96657417111497068, -13.60061260430328467, -3.794707603699265519E-15 ) ) ;
#7584=FACE_OUTER_BOUND ( 'NONE', #8572, .T. ) ;
#7600=EDGE_CURVE ( 'NONE', #988, #8601, #10276, .T. ) ;
#7603=CARTESIAN_POINT ( 'NONE',  ( -16.14082873121598993, -7.414910804916202913, -3.800000000000000266 ) ) ;
#7607=EDGE_CURVE ( 'NONE', #12819, #10457, #12410, .T. ) ;
#7617=CIRCLE ( 'NONE', #7378, 5.000000000000000888 ) ;
#7653=DIRECTION ( 'NONE',  ( -5.480158469902919838E-17, -1.051478716308701618E-16, -1.000000000000000000 ) ) ;
#7656=ORIENTED_EDGE ( 'NONE', *, *, #7607, .F. ) ;
#7659=EDGE_LOOP ( 'NONE', ( #12586, #10041, #13264, #6772 ) ) ;
#7674=EDGE_CURVE ( 'NONE', #1813, #7692, #10447, .T. ) ;
#7691=DIRECTION ( 'NONE',  ( -1.000000000000000000, 0.000000000000000000, 0.000000000000000000 ) ) ;
#7692=VERTEX_POINT ( 'NONE', #7174 ) ;
#7720=AXIS2_PLACEMENT_3D ( 'NONE', #4781, #3688, #3614 ) ;
#7736=CARTESIAN_POINT ( 'NONE',  ( -10.40394475573011945, -10.79473832354794460, -5.000000000000000000 ) ) ;
#7738=LINE ( 'NONE', #11493, #2638 ) ;
#7746=CIRCLE ( 'NONE', #9705, 4.000000000000000000 ) ;
#7750=ORIENTED_EDGE ( 'NONE', *, *, #3195, .F. ) ;
#7751=DIRECTION ( 'NONE',  ( 0.000000000000000000, 0.000000000000000000, 1.000000000000000000 ) ) ;
#7760=DIRECTION ( 'NONE',  ( 1.445602896647338917E-16, -1.000000000000000000, 0.000000000000000000 ) ) ;
#7763=CARTESIAN_POINT ( 'NONE',  ( -14.40394475573011945, -10.79473832354794460, -3.000000000000000000 ) ) ;
#7767=CARTESIAN_POINT ( 'NONE',  ( -10.40394475573011945, -10.79473832354794460, -3.800000000000000266 ) ) ;
#7773=ADVANCED_FACE ( 'NONE', ( #15105 ), #2336, .T. ) ;
#7774=ORIENTED_EDGE ( 'NONE', *, *, #15010, .T. ) ;
#7776=ORIENTED_EDGE ( 'NONE', *, *, #3539, .F. ) ;
#7785=ORIENTED_EDGE ( 'NONE', *, *, #2708, .F. ) ;
#7813=ORIENTED_EDGE ( 'NONE', *, *, #7674, .F. ) ;
#7826=DIRECTION ( 'NONE',  ( 1.576560579138138762E-17, -1.359337748750801762E-17, 1.000000000000000000 ) ) ;
#7837=DIRECTION ( 'NONE',  ( 1.000000000000000000, 1.445602896647338917E-16, -0.000000000000000000 ) ) ;
#7875=ORIENTED_EDGE ( 'NONE', *, *, #13404, .T. ) ;
#7880=EDGE_CURVE ( 'NONE', #12279, #11000, #1490, .T. ) ;
#7884=DIRECTION ( 'NONE',  ( 0.000000000000000000, 1.000000000000000000, -1.084202172485504187E-16 ) ) ;
#7885=CYLINDRICAL_SURFACE ( 'NONE', #13557, 4.000000000000000000 ) ;
#7894=CARTESIAN_POINT ( 'NONE',  ( -16.96657417111497068, -13.60061260430328467, -3.794707603699265519E-15 ) ) ;
#7923=ORIENTED_EDGE ( 'NONE', *, *, #7880, .F. ) ;
#7925=ORIENTED_EDGE ( 'NONE', *, *, #1558, .T. ) ;
#7948=DIRECTION ( 'NONE',  ( -5.480158469902919838E-17, -1.051478716308701618E-16, -1.000000000000000000 ) ) ;
#7960=AXIS2_PLACEMENT_3D ( 'NONE', #10837, #4078, #14303 ) ;
#7965=DIRECTION ( 'NONE',  ( 0.000000000000000000, 1.000000000000000000, 0.000000000000000000 ) ) ;
#7971=AXIS2_PLACEMENT_3D ( 'NONE', #1359, #14206, #10527 ) ;
#7974=CIRCLE ( 'NONE', #1587, 3.799999999999998934 ) ;
#7978=LINE ( 'NONE', #14989, #14136 ) ;
#7980=ORIENTED_EDGE ( 'NONE', *, *, #5458, .F. ) ;
#8024=DIRECTION ( 'NONE',  ( -5.480158469902919838E-17, -1.051478716308701618E-16, -1.000000000000000000 ) ) ;
#8026=EDGE_CURVE ( 'NONE', #1275, #14803, #1817, .T. ) ;
#8036=EDGE_LOOP ( 'NONE', ( #11690, #11703, #14829, #830 ) ) ;
#8081=ORIENTED_EDGE ( 'NONE', *, *, #6384, .T. ) ;
#8097=CARTESIAN_POINT ( 'NONE',  ( -19.40394475573012301, -16.79473832354794993, 16.99999999999999645 ) ) ;
#8102=AXIS2_PLACEMENT_3D ( 'NONE', #13808, #4144, #8817 ) ;
#8106=EDGE_CURVE ( 'NONE', #13077, #12416, #14596, .T. ) ;
#8114=LINE ( 'NONE', #12936, #2659 ) ;
#8149=DIRECTION ( 'NONE',  ( 0.000000000000000000, -1.000000000000000000, 0.000000000000000000 ) ) ;
#8164=EDGE_CURVE ( 'NONE', #1885, #8254, #2571, .T. ) ;
#8172=DIRECTION ( 'NONE',  ( 1.000000000000000000, 0.000000000000000000, 0.000000000000000000 ) ) ;
#8192=DIRECTION ( 'NONE',  ( 1.000000000000000000, 0.000000000000000000, 0.000000000000000000 ) ) ;
#8201=DIRECTION ( 'NONE',  ( -0.4055247608874392173, 0.9140840597599245720, -7.389059384413459453E-17 ) ) ;
#8219=CIRCLE ( 'NONE', #6260, 4.000000000000000000 ) ;
#8254=VERTEX_POINT ( 'NONE', #12527 ) ;
#8257=VECTOR ( 'NONE', #9754, 1000.000000000000000 ) ;
#8265=EDGE_LOOP ( 'NONE', ( #7980, #11453, #11329, #6251 ) ) ;
#8286=CARTESIAN_POINT ( 'NONE',  ( -16.96657417111497068, -13.60061260430328467, 0.7999999999999960476 ) ) ;
#8295=FILL_AREA_STYLE_COLOUR ( '', #11854 ) ;
#8321=ORIENTED_EDGE ( 'NONE', *, *, #15016, .T. ) ;
#8324=CIRCLE ( 'NONE', #6127, 4.000000000000000888 ) ;
#8354=LINE ( 'NONE', #6979, #13426 ) ;
#8372=FACE_OUTER_BOUND ( 'NONE', #14734, .T. ) ;
#8385=ORIENTED_EDGE ( 'NONE', *, *, #14788, .F. ) ;
#8386=VECTOR ( 'NONE', #736, 1000.000000000000000 ) ;
#8429=STYLED_ITEM ( 'NONE', ( #4932 ), #4912 ) ;
#8457=CARTESIAN_POINT ( 'NONE',  ( -14.40394475573012301, -4.794738323547945491, 20.00000000000000000 ) ) ;
#8459=ORIENTED_EDGE ( 'NONE', *, *, #545, .T. ) ;
#8493=PLANE ( 'NONE',  #13921 ) ;
#8515=CARTESIAN_POINT ( 'NONE',  ( -14.40394475573012301, -4.794738323547945491, 16.99999999999999645 ) ) ;
#8572=EDGE_LOOP ( 'NONE', ( #5089, #9102, #7560, #12632 ) ) ;
#8582=CYLINDRICAL_SURFACE ( 'NONE', #13930, 4.000000000000000000 ) ;
#8590=DIRECTION ( 'NONE',  ( -0.000000000000000000, -0.000000000000000000, -1.000000000000000000 ) ) ;
#8596=LINE ( 'NONE', #5080, #8257 ) ;
#8601=VERTEX_POINT ( 'NONE', #4338 ) ;
#8617=ORIENTED_EDGE ( 'NONE', *, *, #6168, .T. ) ;
#8654=CARTESIAN_POINT ( 'NONE',  ( -15.94493884710238696, -7.321218896460230496, -3.000000000000000000 ) ) ;
#8672=DIRECTION ( 'NONE',  ( -1.445602896647338917E-16, 1.000000000000000000, -0.000000000000000000 ) ) ;
#8674=DIRECTION ( 'NONE',  ( 0.8894282943767740646, 0.4570747303910190351, -9.680251508487129501E-17 ) ) ;
#8687=PRODUCT_DEFINITION_CONTEXT ( 'detailed design', #5084, 'design' ) ;
#8690=ORIENTED_EDGE ( 'NONE', *, *, #2708, .T. ) ;
#8700=ORIENTED_EDGE ( 'NONE', *, *, #453, .F. ) ;
#8736=ORIENTED_EDGE ( 'NONE', *, *, #1873, .T. ) ;
#8738=DIRECTION ( 'NONE',  ( 0.000000000000000000, 0.000000000000000000, -1.000000000000000000 ) ) ;
#8740=EDGE_CURVE ( 'NONE', #9424, #7105, #6869, .T. ) ;
#8752=DIRECTION ( 'NONE',  ( 0.000000000000000000, -0.000000000000000000, -1.000000000000000000 ) ) ;
#8773=AXIS2_PLACEMENT_3D ( 'NONE', #5593, #9045, #11411 ) ;
#8779=VERTEX_POINT ( 'NONE', #385 ) ;
#8780=DIRECTION ( 'NONE',  ( 0.7573544145849105957, -0.6530040510661073716, -2.081668171172162967E-17 ) ) ;
#8792=VERTEX_POINT ( 'NONE', #13147 ) ;
#8804=ORIENTED_EDGE ( 'NONE', *, *, #5864, .F. ) ;
#8813=PLANE ( 'NONE',  #2891 ) ;
#8814=DIRECTION ( 'NONE',  ( 0.4570747303910190351, -0.8894282943767740646, 6.847307257068341160E-17 ) ) ;
#8817=DIRECTION ( 'NONE',  ( 0.7573544145849105957, -0.6530040510661073716, -2.081668171172162967E-17 ) ) ;
#8840=DIRECTION ( 'NONE',  ( 0.000000000000000000, 0.000000000000000000, -1.000000000000000000 ) ) ;
#8849=CARTESIAN_POINT ( 'NONE',  ( -10.40394475573011945, -10.79473832354794460, -5.000000000000000000 ) ) ;
#8870=DIRECTION ( 'NONE',  ( 1.000000000000000000, 0.000000000000000000, 0.000000000000000000 ) ) ;
#8897=DIRECTION ( 'NONE',  ( 1.000000000000000000, 0.000000000000000000, -0.000000000000000000 ) ) ;
#8914=DIRECTION ( 'NONE',  ( -0.9140840597599245720, -0.4055247608874392728, 9.273332052389774862E-17 ) ) ;
#8933=AXIS2_PLACEMENT_3D ( 'NONE', #784, #4184, #5493 ) ;
#8940=ORIENTED_EDGE ( 'NONE', *, *, #453, .T. ) ;
#8953=DIRECTION ( 'NONE',  ( -0.6310987668242443727, -0.7757024858236036824, -5.947623346206206400E-19 ) ) ;
#8970=CIRCLE ( 'NONE', #5318, 4.000000000000000000 ) ;
#8985=DIRECTION ( 'NONE',  ( 0.000000000000000000, 0.000000000000000000, 1.000000000000000000 ) ) ;
#9029=EDGE_CURVE ( 'NONE', #13750, #12819, #7058, .T. ) ;
#9033=ORIENTED_EDGE ( 'NONE', *, *, #4019, .F. ) ;
#9045=DIRECTION ( 'NONE',  ( -1.445602896647338917E-16, 1.000000000000000000, -0.000000000000000000 ) ) ;
#9077=ORIENTED_EDGE ( 'NONE', *, *, #12184, .T. ) ;
#9090=ORIENTED_EDGE ( 'NONE', *, *, #140, .F. ) ;
#9102=ORIENTED_EDGE ( 'NONE', *, *, #14959, .T. ) ;
#9131=DIRECTION ( 'NONE',  ( 0.000000000000000000, 0.000000000000000000, 1.000000000000000000 ) ) ;
#9133=EDGE_LOOP ( 'NONE', ( #8700, #10794 ) ) ;
#9136=ORIENTED_EDGE ( 'NONE', *, *, #8106, .T. ) ;
#9160=CARTESIAN_POINT ( 'NONE',  ( -10.97587178374205941, -9.155129925568431304, -3.000000000000000444 ) ) ;
#9162=ORIENTED_EDGE ( 'NONE', *, *, #972, .F. ) ;
#9165=EDGE_CURVE ( 'NONE', #1485, #3479, #13927, .T. ) ;
#9167=ORIENTED_EDGE ( 'NONE', *, *, #4004, .F. ) ;
#9175=( GEOMETRIC_REPRESENTATION_CONTEXT ( 3 ) GLOBAL_UNCERTAINTY_ASSIGNED_CONTEXT ( ( #4094 ) ) GLOBAL_UNIT_ASSIGNED_CONTEXT ( ( #10539, #9312, #14138 ) ) REPRESENTATION_CONTEXT ( 'NONE', 'WORKASPACE' ) );
#9187=EDGE_CURVE ( 'NONE', #12416, #9424, #10978, .T. ) ;
#9189=CARTESIAN_POINT ( 'NONE',  ( -14.40394475573011945, -10.79473832354794283, -3.799999999999999822 ) ) ;
#9197=APPLICATION_CONTEXT ( 'automotive_design' ) ;
#9200=DIRECTION ( 'NONE',  ( 5.782411586589355667E-16, 1.000000000000000000, -0.000000000000000000 ) ) ;
#9209=CARTESIAN_POINT ( 'NONE',  ( -19.40394475573011590, -4.794738323547945491, 16.99999999999999645 ) ) ;
#9211=VERTEX_POINT ( 'NONE', #14298 ) ;
#9231=DIRECTION ( 'NONE',  ( 0.000000000000000000, 0.000000000000000000, -1.000000000000000000 ) ) ;
#9233=EDGE_CURVE ( 'NONE', #12264, #12279, #10770, .T. ) ;
#9237=UNCERTAINTY_MEASURE_WITH_UNIT (LENGTH_MEASURE( 1.000000000000000082E-05 ), #12640, 'distance_accuracy_value', 'NONE');
#9246=CIRCLE ( 'NONE', #14887, 3.799999999999999378 ) ;
#9257=VECTOR ( 'NONE', #4046, 1000.000000000000000 ) ;
#9302=DIRECTION ( 'NONE',  ( 0.000000000000000000, 0.000000000000000000, -1.000000000000000000 ) ) ;
#9312=( NAMED_UNIT ( * ) PLANE_ANGLE_UNIT ( ) SI_UNIT ( $, .RADIAN. ) );
#9331=CARTESIAN_POINT ( 'NONE',  ( -14.40394475573011945, -10.79473832354794460, -3.794707603699265519E-15 ) ) ;
#9338=ORIENTED_EDGE ( 'NONE', *, *, #12382, .T. ) ;
#9341=ORIENTED_EDGE ( 'NONE', *, *, #3195, .T. ) ;
#9347=CARTESIAN_POINT ( 'NONE',  ( -14.40394475573011945, -7.794738323547949044, 22.00000000000000000 ) ) ;
#9367=FACE_OUTER_BOUND ( 'NONE', #3372, .T. ) ;
#9388=CARTESIAN_POINT ( 'NONE',  ( -19.40394475573011590, -4.794738323547945491, 22.00000000000000000 ) ) ;
#9393=DIRECTION ( 'NONE',  ( 0.7573544145849104847, -0.6530040510661075936, -2.081668171172168513E-17 ) ) ;
#9397=DIRECTION ( 'NONE',  ( 0.000000000000000000, 0.000000000000000000, 1.000000000000000000 ) ) ;
#9421=EDGE_CURVE ( 'NONE', #5016, #8792, #13979, .T. ) ;
#9424=VERTEX_POINT ( 'NONE', #10139 ) ;
#9435=VECTOR ( 'NONE', #14245, 1000.000000000000000 ) ;
#9440=DIRECTION ( 'NONE',  ( 1.445602896647338917E-16, -1.000000000000000000, 0.000000000000000000 ) ) ;
#9446=ORIENTED_EDGE ( 'NONE', *, *, #1285, .F. ) ;
#9449=VECTOR ( 'NONE', #4836, 1000.000000000000000 ) ;
#9489=DIRECTION ( 'NONE',  ( -5.480158469902919838E-17, -1.051478716308701618E-16, -1.000000000000000000 ) ) ;
#9498=VECTOR ( 'NONE', #1219, 1000.000000000000000 ) ;
#9502=AXIS2_PLACEMENT_3D ( 'NONE', #14604, #14533, #5090 ) ;
#9512=AXIS2_PLACEMENT_3D ( 'NONE', #6039, #2886, #14423 ) ;
#9560=LINE ( 'NONE', #2491, #7444 ) ;
#9577=VERTEX_POINT ( 'NONE', #6131 ) ;
#9596=CARTESIAN_POINT ( 'NONE',  ( -16.96657417111497068, -13.60061260430328467, -3.794707603699265519E-15 ) ) ;
#9598=DIRECTION ( 'NONE',  ( 0.9021244663126475327, 0.4314758942051350465, -1.141265444721583757E-16 ) ) ;
#9600=ORIENTED_EDGE ( 'NONE', *, *, #1101, .T. ) ;
#9640=DIRECTION ( 'NONE',  ( 1.000000000000000000, 0.000000000000000000, 0.000000000000000000 ) ) ;
#9648=CARTESIAN_POINT ( 'NONE',  ( -18.40394475573011945, -10.79473832354794460, -5.000000000000000000 ) ) ;
#9668=CYLINDRICAL_SURFACE ( 'NONE', #11639, 3.799999999999999378 ) ;
#9678=ORIENTED_EDGE ( 'NONE', *, *, #14913, .T. ) ;
#9691=ORIENTED_EDGE ( 'NONE', *, *, #13890, .F. ) ;
#9705=AXIS2_PLACEMENT_3D ( 'NONE', #1862, #5414, #11001 ) ;
#9714=ORIENTED_EDGE ( 'NONE', *, *, #5817, .F. ) ;
#9715=LINE ( 'NONE', #14412, #5338 ) ;
#9728=CARTESIAN_POINT ( 'NONE',  ( -16.64001273322991281, -13.79473832354794993, 14.99999999999999822 ) ) ;
#9734=CIRCLE ( 'NONE', #7544, 3.799999999999999378 ) ;
#9735=ADVANCED_FACE ( 'NONE', ( #9738 ), #8813, .T. ) ;
#9738=FACE_OUTER_BOUND ( 'NONE', #928, .T. ) ;
#9740=CARTESIAN_POINT ( 'NONE',  ( -18.40394475573011945, -10.79473832354794460, -5.000000000000000000 ) ) ;
#9741=DIRECTION ( 'NONE',  ( -1.445602896647338917E-16, 1.000000000000000000, -0.000000000000000000 ) ) ;
#9754=DIRECTION ( 'NONE',  ( 1.576560579138138762E-17, -1.359337748750801608E-17, 1.000000000000000000 ) ) ;
#9770=ADVANCED_FACE ( 'NONE', ( #14583 ), #4054, .F. ) ;
#9789=EDGE_LOOP ( 'NONE', ( #11095, #1006 ) ) ;
#9794=AXIS2_PLACEMENT_3D ( 'NONE', #3336, #8024, #12706 ) ;
#9849=VERTEX_POINT ( 'NONE', #7894 ) ;
#9884=EDGE_CURVE ( 'NONE', #8779, #15019, #14940, .T. ) ;
#9896=ORIENTED_EDGE ( 'NONE', *, *, #6234, .T. ) ;
#9905=CARTESIAN_POINT ( 'NONE',  ( -19.40394475573011590, -4.794738323547945491, 22.00000000000000000 ) ) ;
#9921=ORIENTED_EDGE ( 'NONE', *, *, #2996, .F. ) ;
#9967=LINE ( 'NONE', #2974, #667 ) ;
#9979=VERTEX_POINT ( 'NONE', #10415 ) ;
#9982=DIRECTION ( 'NONE',  ( -0.000000000000000000, -0.000000000000000000, -1.000000000000000000 ) ) ;
#10037=CARTESIAN_POINT ( 'NONE',  ( -14.40394475573011945, -10.79473832354794283, -3.000000000000000000 ) ) ;
#10041=ORIENTED_EDGE ( 'NONE', *, *, #5323, .T. ) ;
#10044=SHAPE_REPRESENTATION ( 'connector', ( #1376 ), #9175 ) ;
#10069=CARTESIAN_POINT ( 'NONE',  ( -19.40394475573011590, -4.794738323547945491, 22.00000000000000000 ) ) ;
#10075=PLANE ( 'NONE',  #14396 ) ;
#10081=VERTEX_POINT ( 'NONE', #5957 ) ;
#10082=CARTESIAN_POINT ( 'NONE',  ( -17.28189153115278032, -8.313322929496736791, -3.715604213194723273E-15 ) ) ;
#10084=EDGE_CURVE ( 'NONE', #988, #14023, #10639, .T. ) ;
#10092=ADVANCED_FACE ( 'NONE', ( #12254 ), #6115, .F. ) ;
#10103=EDGE_LOOP ( 'NONE', ( #14990, #10844, #358, #834, #14183, #6300, #12661, #1497 ) ) ;
#10139=CARTESIAN_POINT ( 'NONE',  ( -16.80212006966224791, -13.74240776967763900, -3.794707603699265519E-15 ) ) ;
#10140=AXIS2_PLACEMENT_3D ( 'NONE', #11560, #10406, #3710 ) ;
#10148=CARTESIAN_POINT ( 'NONE',  ( -18.40394475573011945, -10.79473832354794460, 0.7999999999999961586 ) ) ;
#10157=DIRECTION ( 'NONE',  ( 0.000000000000000000, 0.000000000000000000, -1.000000000000000000 ) ) ;
#10172=ORIENTED_EDGE ( 'NONE', *, *, #80, .F. ) ;
#10177=ORIENTED_EDGE ( 'NONE', *, *, #2929, .F. ) ;
#10179=DIRECTION ( 'NONE',  ( -0.000000000000000000, -1.000000000000000000, -0.000000000000000000 ) ) ;
#10213=ORIENTED_EDGE ( 'NONE', *, *, #7007, .F. ) ;
#10241=AXIS2_PLACEMENT_3D ( 'NONE', #3213, #968, #5669 ) ;
#10269=ORIENTED_EDGE ( 'NONE', *, *, #4217, .F. ) ;
#10275=CARTESIAN_POINT ( 'NONE',  ( -14.40394475573011945, -10.79473832354794460, 0.7999999999999960476 ) ) ;
#10276=CIRCLE ( 'NONE', #3641, 3.799999999999999378 ) ;
#10290=EDGE_LOOP ( 'NONE', ( #2684, #6808, #9600, #4949 ) ) ;
#10312=VECTOR ( 'NONE', #8590, 1000.000000000000000 ) ;
#10329=ORIENTED_EDGE ( 'NONE', *, *, #7007, .T. ) ;
#10338=EDGE_LOOP ( 'NONE', ( #2585, #10720, #3262, #7222, #6315, #9136, #323, #2796 ) ) ;
#10341=ADVANCED_FACE ( 'NONE', ( #8372 ), #6226, .F. ) ;
#10362=LINE ( 'NONE', #12526, #13848 ) ;
#10371=DIRECTION ( 'NONE',  ( 1.000000000000000000, 1.445602896647338917E-16, -0.000000000000000000 ) ) ;
#10383=VECTOR ( 'NONE', #8953, 1000.000000000000114 ) ;
#10406=DIRECTION ( 'NONE',  ( 1.445602896647338917E-16, -1.000000000000000000, 0.000000000000000000 ) ) ;
#10415=CARTESIAN_POINT ( 'NONE',  ( -9.403944755730119454, -4.794738323547945491, 16.99999999999999645 ) ) ;
#10418=CARTESIAN_POINT ( 'NONE',  ( -14.40394475573011945, -10.79473832354794460, -3.794707603699265519E-15 ) ) ;
#10428=CARTESIAN_POINT ( 'NONE',  ( -14.40394475573011945, -10.79473832354794460, -3.794707603699265519E-15 ) ) ;
#10429=AXIS2_PLACEMENT_3D ( 'NONE', #13341, #9741, #4142 ) ;
#10445=AXIS2_PLACEMENT_3D ( 'NONE', #95, #4971, #12789 ) ;
#10447=CIRCLE ( 'NONE', #1116, 4.000000000000000888 ) ;
#10449=CARTESIAN_POINT ( 'NONE',  ( -16.80212006966224791, -13.74240776967763900, -3.794707603699265519E-15 ) ) ;
#10451=DIRECTION ( 'NONE',  ( 0.9021244663126475327, 0.4314758942051350465, -1.141265444721583757E-16 ) ) ;
#10453=ORIENTED_EDGE ( 'NONE', *, *, #11990, .T. ) ;
#10457=VERTEX_POINT ( 'NONE', #5175 ) ;
#10477=CARTESIAN_POINT ( 'NONE',  ( -16.80212006966224791, -13.74240776967763900, -3.794707603699265519E-15 ) ) ;
#10481=ADVANCED_FACE ( 'NONE', ( #13290, #1926 ), #1621, .F. ) ;
#10483=ORIENTED_EDGE ( 'NONE', *, *, #13966, .F. ) ;
#10514=CARTESIAN_POINT ( 'NONE',  ( 0.000000000000000000, 0.000000000000000000, 12.00000000000000000 ) ) ;
#10527=DIRECTION ( 'NONE',  ( 1.000000000000000000, 0.000000000000000000, 0.000000000000000000 ) ) ;
#10539=( LENGTH_UNIT ( ) NAMED_UNIT ( * ) SI_UNIT ( .MILLI., .METRE. ) );
#10550=CARTESIAN_POINT ( 'NONE',  ( -10.97587178374205941, -9.155129925568431304, -3.800000000000000266 ) ) ;
#10551=AXIS2_PLACEMENT_3D ( 'NONE', #3318, #11311, #14779 ) ;
#10568=EDGE_CURVE ( 'NONE', #12453, #5145, #13363, .T. ) ;
#10581=ORIENTED_EDGE ( 'NONE', *, *, #7322, .T. ) ;
#10589=ADVANCED_FACE ( 'NONE', ( #6454 ), #13593, .T. ) ;
#10602=CARTESIAN_POINT ( 'NONE',  ( -14.40394475573011945, -10.79473832354794283, -3.000000000000000000 ) ) ;
#10604=ORIENTED_EDGE ( 'NONE', *, *, #6634, .T. ) ;
#10607=VERTEX_POINT ( 'NONE', #15143 ) ;
#10618=VERTEX_POINT ( 'NONE', #3379 ) ;
#10639=LINE ( 'NONE', #4815, #14950 ) ;
#10673=EDGE_CURVE ( 'NONE', #10607, #7692, #10362, .T. ) ;
#10720=ORIENTED_EDGE ( 'NONE', *, *, #3944, .T. ) ;
#10727=CARTESIAN_POINT ( 'NONE',  ( -16.14082873121598993, -7.414910804916202913, -3.800000000000000266 ) ) ;
#10739=AXIS2_PLACEMENT_3D ( 'NONE', #10418, #13960, #12788 ) ;
#10770=CIRCLE ( 'NONE', #9502, 3.000000000000000888 ) ;
#10780=ORIENTED_EDGE ( 'NONE', *, *, #12004, .F. ) ;
#10788=EDGE_CURVE ( 'NONE', #12264, #3700, #4757, .T. ) ;
#10794=ORIENTED_EDGE ( 'NONE', *, *, #15016, .F. ) ;
#10802=CARTESIAN_POINT ( 'NONE',  ( -19.40394475573011590, -4.794738323547945491, 12.00000000000000000 ) ) ;
#10811=EDGE_CURVE ( 'NONE', #12279, #2475, #4049, .T. ) ;
#10813=CARTESIAN_POINT ( 'NONE',  ( -14.40394475573012301, -4.794738323547945491, 13.99999999999999645 ) ) ;
#10815=LINE ( 'NONE', #3514, #9498 ) ;
#10837=CARTESIAN_POINT ( 'NONE',  ( -14.40394475573011945, -10.79473832354794460, -3.794707603699265519E-15 ) ) ;
#10844=ORIENTED_EDGE ( 'NONE', *, *, #11140, .F. ) ;
#10878=VERTEX_POINT ( 'NONE', #11113 ) ;
#10881=EDGE_CURVE ( 'NONE', #9577, #8779, #14517, .T. ) ;
#10889=CARTESIAN_POINT ( 'NONE',  ( -9.403944755730117677, -13.79473832354794816, 14.99999999999999822 ) ) ;
#10910=AXIS2_PLACEMENT_3D ( 'NONE', #11127, #7760, #12448 ) ;
#10912=DIRECTION ( 'NONE',  ( 1.000000000000000000, 0.000000000000000000, 2.081668171172168908E-15 ) ) ;
#10923=DIRECTION ( 'NONE',  ( 1.445602896647338917E-16, -1.000000000000000000, 0.000000000000000000 ) ) ;
#10936=EDGE_CURVE ( 'NONE', #10878, #5334, #6997, .T. ) ;
#10965=CIRCLE ( 'NONE', #10241, 3.000000000000000888 ) ;
#10968=CARTESIAN_POINT ( 'NONE',  ( -16.02604379927987566, -7.138402084508245871, -5.000000000000000000 ) ) ;
#10978=CIRCLE ( 'NONE', #10739, 3.799999999999998934 ) ;
#10981=VECTOR ( 'NONE', #11584, 1000.000000000000000 ) ;
#10999=ORIENTED_EDGE ( 'NONE', *, *, #13052, .T. ) ;
#11000=VERTEX_POINT ( 'NONE', #12108 ) ;
#11001=DIRECTION ( 'NONE',  ( -1.000000000000000000, 0.000000000000000000, 0.000000000000000000 ) ) ;
#11009=EDGE_LOOP ( 'NONE', ( #3226, #6722, #6394, #14241 ) ) ;
#11012=DIRECTION ( 'NONE',  ( -5.480158469902919838E-17, -1.051478716308701618E-16, -1.000000000000000000 ) ) ;
#11015=VECTOR ( 'NONE', #3654, 1000.000000000000000 ) ;
#11031=ORIENTED_EDGE ( 'NONE', *, *, #10936, .F. ) ;
#11038=ORIENTED_EDGE ( 'NONE', *, *, #5699, .F. ) ;
#11050=VECTOR ( 'NONE', #9200, 1000.000000000000000 ) ;
#11061=DIRECTION ( 'NONE',  ( -0.000000000000000000, -0.000000000000000000, -1.000000000000000000 ) ) ;
#11070=PLANE ( 'NONE',  #3849 ) ;
#11071=DIRECTION ( 'NONE',  ( 1.000000000000000000, 1.445602896647338917E-16, -0.000000000000000000 ) ) ;
#11081=EDGE_CURVE ( 'NONE', #12694, #1885, #8219, .T. ) ;
#11095=ORIENTED_EDGE ( 'NONE', *, *, #13073, .F. ) ;
#11103=LINE ( 'NONE', #1435, #4408 ) ;
#11113=CARTESIAN_POINT ( 'NONE',  ( -19.40394475573012301, -13.79473832354794993, 16.99999999999999645 ) ) ;
#11127=CARTESIAN_POINT ( 'NONE',  ( -19.40394475573012301, -7.794738323547950820, 16.99999999999999645 ) ) ;
#11140=EDGE_CURVE ( 'NONE', #3735, #14731, #4551, .T. ) ;
#11146=AXIS2_PLACEMENT_3D ( 'NONE', #10069, #2843, #8752 ) ;
#11189=AXIS2_PLACEMENT_3D ( 'NONE', #10602, #7215, #10451 ) ;
#11195=DIRECTION ( 'NONE',  ( 0.000000000000000000, -0.000000000000000000, 1.000000000000000000 ) ) ;
#11198=CYLINDRICAL_SURFACE ( 'NONE', #11735, 5.000000000000000888 ) ;
#11208=ORIENTED_EDGE ( 'NONE', *, *, #3539, .T. ) ;
#11220=ORIENTED_EDGE ( 'NONE', *, *, #10084, .T. ) ;
#11227=EDGE_CURVE ( 'NONE', #9211, #7272, #3496, .T. ) ;
#11229=ORIENTED_EDGE ( 'NONE', *, *, #5864, .T. ) ;
#11237=ADVANCED_FACE ( 'NONE', ( #12863 ), #1200, .T. ) ;
#11247=DIRECTION ( 'NONE',  ( 0.000000000000000000, 0.000000000000000000, 1.000000000000000000 ) ) ;
#11261=CARTESIAN_POINT ( 'NONE',  ( -14.40394475573011945, -10.79473832354794283, -3.000000000000000000 ) ) ;
#11274=DIRECTION ( 'NONE',  ( 1.000000000000000000, 0.000000000000000000, -2.710505431213761085E-17 ) ) ;
#11283=DIRECTION ( 'NONE',  ( 1.576560579138138762E-17, -1.359337748750801608E-17, 1.000000000000000000 ) ) ;
#11288=LINE ( 'NONE', #3068, #4073 ) ;
#11302=DIRECTION ( 'NONE',  ( 0.000000000000000000, 0.000000000000000000, -1.000000000000000000 ) ) ;
#11311=DIRECTION ( 'NONE',  ( 5.782411586589355667E-16, 1.000000000000000000, 0.000000000000000000 ) ) ;
#11329=ORIENTED_EDGE ( 'NONE', *, *, #6384, .F. ) ;
#11349=FACE_OUTER_BOUND ( 'NONE', #12773, .T. ) ;
#11386=AXIS2_PLACEMENT_3D ( 'NONE', #5883, #9397, #7020 ) ;
#11401=ORIENTED_EDGE ( 'NONE', *, *, #5060, .F. ) ;
#11411=DIRECTION ( 'NONE',  ( 1.000000000000000000, 1.734723475976807341E-16, -6.938893903907229364E-16 ) ) ;
#11413=CARTESIAN_POINT ( 'NONE',  ( -10.40394475573011945, -10.79473832354794460, -5.000000000000000000 ) ) ;
#11425=ORIENTED_EDGE ( 'NONE', *, *, #11227, .F. ) ;
#11428=ORIENTED_EDGE ( 'NONE', *, *, #13871, .F. ) ;
#11445=DIRECTION ( 'NONE',  ( 1.000000000000000000, 0.000000000000000000, 0.000000000000000000 ) ) ;
#11453=ORIENTED_EDGE ( 'NONE', *, *, #1399, .F. ) ;
#11488=ORIENTED_EDGE ( 'NONE', *, *, #11950, .F. ) ;
#11493=CARTESIAN_POINT ( 'NONE',  ( -11.52599798030746037, -13.27615371759915242, -3.873810994203807765E-15 ) ) ;
#11503=ORIENTED_EDGE ( 'NONE', *, *, #5817, .T. ) ;
#11547=ADVANCED_FACE ( 'NONE', ( #5799 ), #4655, .T. ) ;
#11556=FACE_OUTER_BOUND ( 'NONE', #7659, .T. ) ;
#11560=CARTESIAN_POINT ( 'NONE',  ( -14.40394475573012301, -7.794738323547949932, 16.99999999999999645 ) ) ;
#11575=CARTESIAN_POINT ( 'NONE',  ( -17.28189153115278032, -8.313322929496736791, -3.715604213194723273E-15 ) ) ;
#11579=DIRECTION ( 'NONE',  ( -0.000000000000000000, -0.000000000000000000, -1.000000000000000000 ) ) ;
#11584=DIRECTION ( 'NONE',  ( -1.445602896647338917E-16, 1.000000000000000000, -0.000000000000000000 ) ) ;
#11594=DIRECTION ( 'NONE',  ( 0.9021244663126475327, 0.4314758942051350465, -1.141265444721583757E-16 ) ) ;
#11627=VECTOR ( 'NONE', #699, 1000.000000000000000 ) ;
#11639=AXIS2_PLACEMENT_3D ( 'NONE', #14369, #3832, #9598 ) ;
#11644=ORIENTED_EDGE ( 'NONE', *, *, #1873, .F. ) ;
#11662=DIRECTION ( 'NONE',  ( 1.576560579138138762E-17, -1.359337748750801608E-17, 1.000000000000000000 ) ) ;
#11664=ADVANCED_FACE ( 'NONE', ( #11917 ), #6097, .T. ) ;
#11667=PLANE ( 'NONE',  #14855 ) ;
#11682=ORIENTED_EDGE ( 'NONE', *, *, #1846, .T. ) ;
#11690=ORIENTED_EDGE ( 'NONE', *, *, #8106, .F. ) ;
#11692=AXIS2_PLACEMENT_3D ( 'NONE', #12501, #1975, #6659 ) ;
#11703=ORIENTED_EDGE ( 'NONE', *, *, #3517, .T. ) ;
#11727=ORIENTED_EDGE ( 'NONE', *, *, #12004, .T. ) ;
#11735=AXIS2_PLACEMENT_3D ( 'NONE', #13884, #6742, #819 ) ;
#11738=ADVANCED_FACE ( 'NONE', ( #13237 ), #2717, .F. ) ;
#11751=AXIS2_PLACEMENT_3D ( 'NONE', #12923, #3482, #8172 ) ;
#11793=DIRECTION ( 'NONE',  ( -5.480158469902919838E-17, -1.051478716308701618E-16, -1.000000000000000000 ) ) ;
#11840=ORIENTED_EDGE ( 'NONE', *, *, #1558, .F. ) ;
#11851=ORIENTED_EDGE ( 'NONE', *, *, #13871, .T. ) ;
#11854=COLOUR_RGB ( '',0.8941176470588234615, 0.8941176470588234615, 0.8941176470588234615 ) ;
#11873=ORIENTED_EDGE ( 'NONE', *, *, #14823, .T. ) ;
#11893=ORIENTED_EDGE ( 'NONE', *, *, #80, .T. ) ;
#11911=DIRECTION ( 'NONE',  ( 1.000000000000000000, -5.782411586589355667E-16, 0.000000000000000000 ) ) ;
#11917=FACE_OUTER_BOUND ( 'NONE', #7401, .T. ) ;
#11925=ORIENTED_EDGE ( 'NONE', *, *, #6331, .T. ) ;
#11950=EDGE_CURVE ( 'NONE', #2971, #9211, #12286, .T. ) ;
#11951=ORIENTED_EDGE ( 'NONE', *, *, #5713, .F. ) ;
#11952=AXIS2_PLACEMENT_3D ( 'NONE', #9189, #6591, #2118 ) ;
#11963=LINE ( 'NONE', #10968, #10312 ) ;
#11970=ORIENTED_EDGE ( 'NONE', *, *, #5060, .T. ) ;
#11978=CLOSED_SHELL ( 'NONE', ( #3275, #6572, #6079, #650, #2113, #6612, #13785, #7773, #2620, #12301, #7228, #5248, #9735, #11738, #10481, #12829, #6006, #3563, #11237, #11664, #3732, #3252, #10589, #9770, #10092, #725, #11547, #6021, #532, #1722, #1882, #1809, #10341, #2703 ) ) ;
#11985=CIRCLE ( 'NONE', #5392, 3.799999999999998934 ) ;
#11990=EDGE_CURVE ( 'NONE', #5125, #12375, #11288, .T. ) ;
#11992=ORIENTED_EDGE ( 'NONE', *, *, #13229, .F. ) ;
#12004=EDGE_CURVE ( 'NONE', #9979, #10618, #7978, .T. ) ;
#12015=ORIENTED_EDGE ( 'NONE', *, *, #1543, .T. ) ;
#12022=LINE ( 'NONE', #8849, #11015 ) ;
#12050=VERTEX_POINT ( 'NONE', #4524 ) ;
#12101=EDGE_LOOP ( 'NONE', ( #2027, #14391, #11893, #9678, #8736, #880, #1022, #14762 ) ) ;
#12108=CARTESIAN_POINT ( 'NONE',  ( -14.40394475573012301, -16.79473832354794993, 20.00000000000000000 ) ) ;
#12115=LINE ( 'NONE', #2688, #5372 ) ;
#12182=ORIENTED_EDGE ( 'NONE', *, *, #1259, .F. ) ;
#12184=EDGE_CURVE ( 'NONE', #12375, #2475, #1529, .T. ) ;
#12194=VECTOR ( 'NONE', #12271, 1000.000000000000000 ) ;
#12200=AXIS2_PLACEMENT_3D ( 'NONE', #5887, #1111, #14021 ) ;
#12254=FACE_OUTER_BOUND ( 'NONE', #14139, .T. ) ;
#12264=VERTEX_POINT ( 'NONE', #4523 ) ;
#12268=ORIENTED_EDGE ( 'NONE', *, *, #1399, .T. ) ;
#12270=DIRECTION ( 'NONE',  ( 0.000000000000000000, 0.000000000000000000, -1.000000000000000000 ) ) ;
#12271=DIRECTION ( 'NONE',  ( 0.000000000000000000, 0.000000000000000000, 1.000000000000000000 ) ) ;
#12279=VERTEX_POINT ( 'NONE', #5461 ) ;
#12286=LINE ( 'NONE', #1760, #14879 ) ;
#12294=DIRECTION ( 'NONE',  ( 1.000000000000000000, 0.000000000000000000, -2.710505431213761085E-17 ) ) ;
#12301=ADVANCED_FACE ( 'NONE', ( #3223 ), #13586, .T. ) ;
#12309=ORIENTED_EDGE ( 'NONE', *, *, #14650, .T. ) ;
#12310=CARTESIAN_POINT ( 'NONE',  ( -19.40394475573011590, -4.794738323547945491, 16.99999999999999645 ) ) ;
#12339=CARTESIAN_POINT ( 'NONE',  ( -14.40394475573011945, -10.79473832354794460, -5.000000000000000000 ) ) ;
#12367=ORIENTED_EDGE ( 'NONE', *, *, #14823, .F. ) ;
#12375=VERTEX_POINT ( 'NONE', #1834 ) ;
#12382=EDGE_CURVE ( 'NONE', #9979, #7272, #1058, .T. ) ;
#12410=LINE ( 'NONE', #3264, #14381 ) ;
#12416=VERTEX_POINT ( 'NONE', #6255 ) ;
#12447=CARTESIAN_POINT ( 'NONE',  ( -17.28189153115278032, -8.313322929496736791, 0.7999999999999961586 ) ) ;
#12448=DIRECTION ( 'NONE',  ( 1.000000000000000000, 1.445602896647338917E-16, 0.000000000000000000 ) ) ;
#12453=VERTEX_POINT ( 'NONE', #9209 ) ;
#12454=DIRECTION ( 'NONE',  ( -0.4055247608874392173, 0.9140840597599244610, -7.389059384413458221E-17 ) ) ;
#12493=AXIS2_PLACEMENT_3D ( 'NONE', #49, #11662, #12815 ) ;
#12497=VERTEX_POINT ( 'NONE', #3793 ) ;
#12501=CARTESIAN_POINT ( 'NONE',  ( -14.40394475573011945, -10.79473832354794460, -3.000000000000000000 ) ) ;
#12505=( NAMED_UNIT ( * ) SI_UNIT ( $, .STERADIAN. ) SOLID_ANGLE_UNIT ( ) );
#12507=DIRECTION ( 'NONE',  ( -5.480158469902919838E-17, -1.051478716308701618E-16, -1.000000000000000000 ) ) ;
#12514=CARTESIAN_POINT ( 'NONE',  ( -16.02604379927987566, -7.138402084508245871, -3.800000000000000266 ) ) ;
#12524=EDGE_LOOP ( 'NONE', ( #4944, #194, #983, #8804 ) ) ;
#12526=CARTESIAN_POINT ( 'NONE',  ( -18.40394475573011945, -10.79473832354794460, -5.000000000000000000 ) ) ;
#12527=CARTESIAN_POINT ( 'NONE',  ( -17.10144940350364706, -13.74829019802725050, 0.7999999999999960476 ) ) ;
#12536=ORIENTED_EDGE ( 'NONE', *, *, #9421, .F. ) ;
#12544=DIRECTION ( 'NONE',  ( -1.445602896647338917E-16, 1.000000000000000000, -0.000000000000000000 ) ) ;
#12553=EDGE_CURVE ( 'NONE', #7105, #12050, #9715, .T. ) ;
#12561=CARTESIAN_POINT ( 'NONE',  ( -14.40394475573011945, -10.79473832354794460, -5.000000000000000000 ) ) ;
#12586=ORIENTED_EDGE ( 'NONE', *, *, #1967, .F. ) ;
#12622=ORIENTED_EDGE ( 'NONE', *, *, #10568, .T. ) ;
#12631=CYLINDRICAL_SURFACE ( 'NONE', #14796, 3.799999999999999378 ) ;
#12632=ORIENTED_EDGE ( 'NONE', *, *, #3417, .F. ) ;
#12640=( LENGTH_UNIT ( ) NAMED_UNIT ( * ) SI_UNIT ( .MILLI., .METRE. ) );
#12648=CARTESIAN_POINT ( 'NONE',  ( -9.403944755730119454, -4.794738323547945491, 12.00000000000000000 ) ) ;
#12661=ORIENTED_EDGE ( 'NONE', *, *, #11081, .F. ) ;
#12680=ORIENTED_EDGE ( 'NONE', *, *, #29, .T. ) ;
#12694=VERTEX_POINT ( 'NONE', #4650 ) ;
#12699=VERTEX_POINT ( 'NONE', #8097 ) ;
#12706=DIRECTION ( 'NONE',  ( 0.9021244663126475327, 0.4314758942051350465, -1.141265444721583757E-16 ) ) ;
#12744=EDGE_CURVE ( 'NONE', #10607, #6338, #8970, .T. ) ;
#12746=PLANE ( 'NONE',  #4902 ) ;
#12773=EDGE_LOOP ( 'NONE', ( #12536, #5531, #10780, #9714 ) ) ;
#12788=DIRECTION ( 'NONE',  ( 0.7573544145849105957, -0.6530040510661073716, -2.081668171172162967E-17 ) ) ;
#12789=DIRECTION ( 'NONE',  ( 1.000000000000000000, 1.445602896647338424E-16, 0.000000000000000000 ) ) ;
#12814=CARTESIAN_POINT ( 'NONE',  ( -14.40394475573012301, -4.794738323547945491, 16.99999999999999645 ) ) ;
#12815=DIRECTION ( 'NONE',  ( 0.7573544145849105957, -0.6530040510661073716, -2.081668171172162967E-17 ) ) ;
#12819=VERTEX_POINT ( 'NONE', #8457 ) ;
#12829=ADVANCED_FACE ( 'NONE', ( #14076 ), #14238, .F. ) ;
#12856=DIRECTION ( 'NONE',  ( -0.000000000000000000, -1.000000000000000000, -0.000000000000000000 ) ) ;
#12863=FACE_OUTER_BOUND ( 'NONE', #8265, .T. ) ;
#12880=DIRECTION ( 'NONE',  ( 1.445602896647338917E-16, -1.000000000000000000, -0.000000000000000000 ) ) ;
#12887=ORIENTED_EDGE ( 'NONE', *, *, #14741, .F. ) ;
#12923=CARTESIAN_POINT ( 'NONE',  ( -14.40394475573011945, -10.79473832354794460, -5.000000000000000000 ) ) ;
#12936=CARTESIAN_POINT ( 'NONE',  ( -14.40394475573012301, -4.794738323547945491, 13.99999999999999645 ) ) ;
#12947=ORIENTED_EDGE ( 'NONE', *, *, #13073, .T. ) ;
#12955=ORIENTED_EDGE ( 'NONE', *, *, #3517, .F. ) ;
#12962=LINE ( 'NONE', #13106, #6564 ) ;
#12967=CARTESIAN_POINT ( 'NONE',  ( -14.40394475573011945, -4.794738323547945491, 16.99999999999999645 ) ) ;
#12976=SURFACE_STYLE_FILL_AREA ( #1076 ) ;
#12977=ORIENTED_EDGE ( 'NONE', *, *, #11950, .T. ) ;
#12999=CARTESIAN_POINT ( 'NONE',  ( -14.40394475573011768, -16.79473832354794993, 22.00000000000000000 ) ) ;
#13021=CYLINDRICAL_SURFACE ( 'NONE', #1945, 3.799999999999998934 ) ;
#13052=EDGE_CURVE ( 'NONE', #761, #14623, #1619, .T. ) ;
#13055=LINE ( 'NONE', #5018, #5820 ) ;
#13062=ORIENTED_EDGE ( 'NONE', *, *, #10673, .F. ) ;
#13066=CARTESIAN_POINT ( 'NONE',  ( -14.40394475573011768, -7.794738323547949932, 16.99999999999999645 ) ) ;
#13073=EDGE_CURVE ( 'NONE', #14059, #13883, #7746, .T. ) ;
#13077=VERTEX_POINT ( 'NONE', #10082 ) ;
#13085=DIRECTION ( 'NONE',  ( 0.4570747303910190351, -0.8894282943767740646, 6.847307257068341160E-17 ) ) ;
#13088=CIRCLE ( 'NONE', #6735, 4.000000000000000000 ) ;
#13106=CARTESIAN_POINT ( 'NONE',  ( -15.94493884710238696, -7.321218896460230496, -3.800000000000000266 ) ) ;
#13115=VECTOR ( 'NONE', #13470, 1000.000000000000000 ) ;
#13117=ORIENTED_EDGE ( 'NONE', *, *, #10811, .T. ) ;
#13141=CARTESIAN_POINT ( 'NONE',  ( -14.40394475573011945, -10.79473832354794283, -3.799999999999999822 ) ) ;
#13142=AXIS2_PLACEMENT_3D ( 'NONE', #7406, #6241, #10923 ) ;
#13147=CARTESIAN_POINT ( 'NONE',  ( -14.40394475573011945, -4.794738323547945491, 22.00000000000000000 ) ) ;
#13156=LINE ( 'NONE', #162, #4409 ) ;
#13201=DIRECTION ( 'NONE',  ( 1.000000000000000000, 0.000000000000000000, -1.576560579138137530E-17 ) ) ;
#13229=EDGE_CURVE ( 'NONE', #6338, #10607, #5100, .T. ) ;
#13237=FACE_OUTER_BOUND ( 'NONE', #2297, .T. ) ;
#13253=AXIS2_PLACEMENT_3D ( 'NONE', #6670, #7826, #5603 ) ;
#13264=ORIENTED_EDGE ( 'NONE', *, *, #9165, .T. ) ;
#13266=DIRECTION ( 'NONE',  ( 1.000000000000000000, 0.000000000000000000, 0.000000000000000000 ) ) ;
#13290=FACE_BOUND ( 'NONE', #13769, .T. ) ;
#13293=ORIENTED_EDGE ( 'NONE', *, *, #5081, .T. ) ;
#13341=CARTESIAN_POINT ( 'NONE',  ( -14.40394475573012123, -13.79473832354794993, 16.99999999999999645 ) ) ;
#13359=ORIENTED_EDGE ( 'NONE', *, *, #7322, .F. ) ;
#13363=LINE ( 'NONE', #9905, #1091 ) ;
#13387=LINE ( 'NONE', #12310, #13115 ) ;
#13399=ORIENTED_EDGE ( 'NONE', *, *, #9029, .T. ) ;
#13404=EDGE_CURVE ( 'NONE', #8254, #14803, #6302, .T. ) ;
#13421=CARTESIAN_POINT ( 'NONE',  ( -14.40394475573012301, -4.794738323547945491, 16.99999999999999645 ) ) ;
#13426=VECTOR ( 'NONE', #12880, 1000.000000000000000 ) ;
#13470=DIRECTION ( 'NONE',  ( 5.782411586589355667E-16, 1.000000000000000000, -0.000000000000000000 ) ) ;
#13494=ORIENTED_EDGE ( 'NONE', *, *, #12184, .F. ) ;
#13496=CARTESIAN_POINT ( 'NONE',  ( -19.40394475573012301, -7.794738323547950820, 14.99999999999999822 ) ) ;
#13509=PRODUCT ( 'connector', 'connector', '', ( #13576 ) ) ;
#13510=CARTESIAN_POINT ( 'NONE',  ( -19.40394475573012301, -16.79473832354794993, 22.00000000000000000 ) ) ;
#13557=AXIS2_PLACEMENT_3D ( 'NONE', #12561, #4201, #8870 ) ;
#13576=PRODUCT_CONTEXT ( 'NONE', #9197, 'mechanical' ) ;
#13586=PLANE ( 'NONE',  #2608 ) ;
#13593=PLANE ( 'NONE',  #10910 ) ;
#13604=CIRCLE ( 'NONE', #14588, 5.000000000000000888 ) ;
#13629=ORIENTED_EDGE ( 'NONE', *, *, #5323, .F. ) ;
#13634=SHAPE_REPRESENTATION_RELATIONSHIP ( 'NONE' , 'NONE' ,  #10044, #4912 ) ;
#13646=EDGE_LOOP ( 'NONE', ( #1025, #5106, #10581, #3779, #10172, #11873, #1129, #69, #3578, #11229, #6994, #14505 ) ) ;
#13648=DIRECTION ( 'NONE',  ( 0.000000000000000000, 0.000000000000000000, 1.000000000000000000 ) ) ;
#13669=CIRCLE ( 'NONE', #7086, 3.000000000000000888 ) ;
#13707=CARTESIAN_POINT ( 'NONE',  ( -19.40394475573012301, -7.794738323547950820, 14.99999999999999822 ) ) ;
#13711=ORIENTED_EDGE ( 'NONE', *, *, #14741, .T. ) ;
#13734=CARTESIAN_POINT ( 'NONE',  ( -14.40394475573011945, -10.79473832354794460, -3.000000000000000000 ) ) ;
#13736=DIRECTION ( 'NONE',  ( 1.576560579138138762E-17, -1.359337748750801608E-17, 1.000000000000000000 ) ) ;
#13739=FACE_OUTER_BOUND ( 'NONE', #8036, .T. ) ;
#13750=VERTEX_POINT ( 'NONE', #10813 ) ;
#13762=CARTESIAN_POINT ( 'NONE',  ( -19.40394475573012301, -7.794738323547950820, 14.99999999999999822 ) ) ;
#13769=EDGE_LOOP ( 'NONE', ( #13399, #2899 ) ) ;
#13785=ADVANCED_FACE ( 'NONE', ( #5294 ), #8582, .T. ) ;
#13808=CARTESIAN_POINT ( 'NONE',  ( -14.40394475573011945, -10.79473832354794460, -3.794707603699265519E-15 ) ) ;
#13829=PLANE ( 'NONE',  #7530 ) ;
#13848=VECTOR ( 'NONE', #8985, 1000.000000000000000 ) ;
#13871=EDGE_CURVE ( 'NONE', #14210, #5016, #6811, .T. ) ;
#13877=DIRECTION ( 'NONE',  ( 0.000000000000000000, 0.000000000000000000, 1.000000000000000000 ) ) ;
#13883=VERTEX_POINT ( 'NONE', #3211 ) ;
#13884=CARTESIAN_POINT ( 'NONE',  ( -14.40394475573011945, -2.082238426203170629E-15, 16.99999999999999645 ) ) ;
#13888=EDGE_CURVE ( 'NONE', #15019, #3945, #4210, .T. ) ;
#13890=EDGE_CURVE ( 'NONE', #14023, #1485, #15166, .T. ) ;
#13907=ORIENTED_EDGE ( 'NONE', *, *, #11227, .T. ) ;
#13909=CARTESIAN_POINT ( 'NONE',  ( -14.40394475573011945, -10.79473832354794283, -3.000000000000000000 ) ) ;
#13919=ORIENTED_EDGE ( 'NONE', *, *, #9233, .T. ) ;
#13920=DIRECTION ( 'NONE',  ( -1.000000000000000000, 0.000000000000000000, 0.000000000000000000 ) ) ;
#13921=AXIS2_PLACEMENT_3D ( 'NONE', #13496, #14431, #417 ) ;
#13927=CIRCLE ( 'NONE', #3866, 3.799999999999999378 ) ;
#13930=AXIS2_PLACEMENT_3D ( 'NONE', #7368, #5066, #13266 ) ;
#13940=MANIFOLD_SOLID_BREP ( 'Cavity1', #11978 ) ;
#13957=ORIENTED_EDGE ( 'NONE', *, *, #2996, .T. ) ;
#13960=DIRECTION ( 'NONE',  ( -1.576560579138138762E-17, 1.359337748750801608E-17, -1.000000000000000000 ) ) ;
#13966=EDGE_CURVE ( 'NONE', #13750, #2791, #8114, .T. ) ;
#13968=DIRECTION ( 'NONE',  ( 0.7573544145849105957, -0.6530040510661073716, -2.853163611803960010E-17 ) ) ;
#13979=LINE ( 'NONE', #3156, #10981 ) ;
#13991=CARTESIAN_POINT ( 'NONE',  ( -14.40394475573011590, -4.794738323547945491, 16.99999999999999645 ) ) ;
#14021=DIRECTION ( 'NONE',  ( 1.000000000000000000, 0.000000000000000000, -1.576560579138137530E-17 ) ) ;
#14022=LINE ( 'NONE', #3564, #5827 ) ;
#14023=VERTEX_POINT ( 'NONE', #3569 ) ;
#14034=CARTESIAN_POINT ( 'NONE',  ( -14.40394475573011945, -10.79473832354794460, -3.799999999999999822 ) ) ;
#14051=DIRECTION ( 'NONE',  ( -0.6310987668242443727, -0.7757024858236036824, -5.947623346206206400E-19 ) ) ;
#14057=( NAMED_UNIT ( * ) PLANE_ANGLE_UNIT ( ) SI_UNIT ( $, .RADIAN. ) );
#14059=VERTEX_POINT ( 'NONE', #2797 ) ;
#14071=ORIENTED_EDGE ( 'NONE', *, *, #10788, .T. ) ;
#14076=FACE_OUTER_BOUND ( 'NONE', #6993, .T. ) ;
#14106=CARTESIAN_POINT ( 'NONE',  ( -15.94493884710238696, -7.321218896460230496, -3.000000000000000000 ) ) ;
#14116=ORIENTED_EDGE ( 'NONE', *, *, #6724, .F. ) ;
#14136=VECTOR ( 'NONE', #14760, 1000.000000000000000 ) ;
#14138=( NAMED_UNIT ( * ) SI_UNIT ( $, .STERADIAN. ) SOLID_ANGLE_UNIT ( ) );
#14139=EDGE_LOOP ( 'NONE', ( #12015, #10213, #276, #1909 ) ) ;
#14156=AXIS2_PLACEMENT_3D ( 'NONE', #10514, #5967, #8192 ) ;
#14158=ORIENTED_EDGE ( 'NONE', *, *, #7880, .T. ) ;
#14169=LINE ( 'NONE', #2719, #9435 ) ;
#14180=CIRCLE ( 'NONE', #9512, 4.000000000000000000 ) ;
#14181=ORIENTED_EDGE ( 'NONE', *, *, #10568, .F. ) ;
#14183=ORIENTED_EDGE ( 'NONE', *, *, #1543, .F. ) ;
#14190=VECTOR ( 'NONE', #7294, 1000.000000000000000 ) ;
#14206=DIRECTION ( 'NONE',  ( 1.445602896647338917E-16, -1.000000000000000000, 0.000000000000000000 ) ) ;
#14210=VERTEX_POINT ( 'NONE', #2243 ) ;
#14238=PLANE ( 'NONE',  #3567 ) ;
#14241=ORIENTED_EDGE ( 'NONE', *, *, #5081, .F. ) ;
#14245=DIRECTION ( 'NONE',  ( -1.445602896647338917E-16, 1.000000000000000000, 0.000000000000000000 ) ) ;
#14298=CARTESIAN_POINT ( 'NONE',  ( -9.403944755730117677, -16.79473832354794993, 12.00000000000000000 ) ) ;
#14303=DIRECTION ( 'NONE',  ( 0.7573544145849105957, -0.6530040510661073716, -2.081668171172162967E-17 ) ) ;
#14356=CARTESIAN_POINT ( 'NONE',  ( -16.80212006966224791, -13.74240776967763900, 0.7999999999999960476 ) ) ;
#14369=CARTESIAN_POINT ( 'NONE',  ( -14.40394475573011945, -10.79473832354794283, -3.000000000000000000 ) ) ;
#14374=ORIENTED_EDGE ( 'NONE', *, *, #7049, .T. ) ;
#14378=DIRECTION ( 'NONE',  ( 5.480158469902919838E-17, 1.051478716308701618E-16, 1.000000000000000000 ) ) ;
#14381=VECTOR ( 'NONE', #4200, 1000.000000000000000 ) ;
#14391=ORIENTED_EDGE ( 'NONE', *, *, #5699, .T. ) ;
#14396=AXIS2_PLACEMENT_3D ( 'NONE', #4238, #8914, #12454 ) ;
#14412=CARTESIAN_POINT ( 'NONE',  ( -16.92833982302709828, -13.89754826684236022, -5.000000000000000000 ) ) ;
#14423=DIRECTION ( 'NONE',  ( 1.000000000000000000, 0.000000000000000000, -2.710505431213761085E-17 ) ) ;
#14431=DIRECTION ( 'NONE',  ( 0.000000000000000000, 0.000000000000000000, 1.000000000000000000 ) ) ;
#14440=DIRECTION ( 'NONE',  ( 0.000000000000000000, 0.000000000000000000, -1.000000000000000000 ) ) ;
#14447=DIRECTION ( 'NONE',  ( 1.576560579138138762E-17, -1.359337748750801608E-17, 1.000000000000000000 ) ) ;
#14460=ORIENTED_EDGE ( 'NONE', *, *, #11990, .F. ) ;
#14467=CARTESIAN_POINT ( 'NONE',  ( -14.40394475573011945, -10.79473832354794460, 0.7999999999999960476 ) ) ;
#14472=CIRCLE ( 'NONE', #7059, 4.000000000000000888 ) ;
#14477=VERTEX_POINT ( 'NONE', #5174 ) ;
#14485=DIRECTION ( 'NONE',  ( -1.000000000000000000, 5.782411586589353694E-16, 0.000000000000000000 ) ) ;
#14505=ORIENTED_EDGE ( 'NONE', *, *, #15010, .F. ) ;
#14517=LINE ( 'NONE', #8654, #3077 ) ;
#14525=CYLINDRICAL_SURFACE ( 'NONE', #387, 3.000000000000000888 ) ;
#14533=DIRECTION ( 'NONE',  ( 1.445602896647338917E-16, -1.000000000000000000, 0.000000000000000000 ) ) ;
#14566=ORIENTED_EDGE ( 'NONE', *, *, #6391, .F. ) ;
#14583=FACE_OUTER_BOUND ( 'NONE', #3941, .T. ) ;
#14588=AXIS2_PLACEMENT_3D ( 'NONE', #5802, #2332, #3141 ) ;
#14596=CIRCLE ( 'NONE', #7960, 3.799999999999998934 ) ;
#14604=CARTESIAN_POINT ( 'NONE',  ( -14.40394475573012301, -13.79473832354794993, 16.99999999999999645 ) ) ;
#14623=VERTEX_POINT ( 'NONE', #12447 ) ;
#14650=EDGE_CURVE ( 'NONE', #418, #2971, #8354, .T. ) ;
#14653=CARTESIAN_POINT ( 'NONE',  ( -19.40394475573012301, -16.79473832354794993, 22.00000000000000000 ) ) ;
#14656=CARTESIAN_POINT ( 'NONE',  ( -19.40394475573011590, -4.794738323547945491, 12.00000000000000000 ) ) ;
#14668=LINE ( 'NONE', #9740, #12194 ) ;
#14731=VERTEX_POINT ( 'NONE', #14356 ) ;
#14734=EDGE_LOOP ( 'NONE', ( #8385, #7169, #9691, #11840, #11401, #13359, #7813, #14566 ) ) ;
#14736=CARTESIAN_POINT ( 'NONE',  ( -16.80212006966224791, -13.74240776967763900, 0.7999999999999960476 ) ) ;
#14741=EDGE_CURVE ( 'NONE', #14210, #5125, #10815, .T. ) ;
#14742=ORIENTED_EDGE ( 'NONE', *, *, #972, .T. ) ;
#14760=DIRECTION ( 'NONE',  ( 1.445602896647338917E-16, -1.000000000000000000, -0.000000000000000000 ) ) ;
#14762=ORIENTED_EDGE ( 'NONE', *, *, #10881, .T. ) ;
#14771=CARTESIAN_POINT ( 'NONE',  ( -14.40394475573011945, -10.79473832354794283, -3.000000000000000000 ) ) ;
#14779=DIRECTION ( 'NONE',  ( -1.000000000000000000, 5.782411586589353694E-16, 0.000000000000000000 ) ) ;
#14788=EDGE_CURVE ( 'NONE', #3479, #2220, #12962, .T. ) ;
#14796=AXIS2_PLACEMENT_3D ( 'NONE', #10037, #7948, #1973 ) ;
#14802=FACE_OUTER_BOUND ( 'NONE', #15000, .T. ) ;
#14803=VERTEX_POINT ( 'NONE', #5974 ) ;
#14808=ORIENTED_EDGE ( 'NONE', *, *, #12553, .T. ) ;
#14823=EDGE_CURVE ( 'NONE', #14477, #1275, #14668, .T. ) ;
#14829=ORIENTED_EDGE ( 'NONE', *, *, #7383, .T. ) ;
#14855=AXIS2_PLACEMENT_3D ( 'NONE', #5923, #9440, #7298 ) ;
#14856=CYLINDRICAL_SURFACE ( 'NONE', #10551, 5.000000000000000888 ) ;
#14865=DIRECTION ( 'NONE',  ( -1.000000000000000000, 0.000000000000000000, 0.000000000000000000 ) ) ;
#14872=ORIENTED_EDGE ( 'NONE', *, *, #9233, .F. ) ;
#14873=CARTESIAN_POINT ( 'NONE',  ( -14.40394475573011945, -10.79473832354794460, -3.799999999999999822 ) ) ;
#14879=VECTOR ( 'NONE', #9982, 1000.000000000000000 ) ;
#14887=AXIS2_PLACEMENT_3D ( 'NONE', #13909, #6917, #11594 ) ;
#14913=EDGE_CURVE ( 'NONE', #12497, #3107, #9967, .T. ) ;
#14940=CIRCLE ( 'NONE', #3626, 4.000000000000000888 ) ;
#14950=VECTOR ( 'NONE', #9489, 1000.000000000000000 ) ;
#14959=EDGE_CURVE ( 'NONE', #12416, #3735, #7738, .T. ) ;
#14963=AXIS2_PLACEMENT_3D ( 'NONE', #6492, #10179, #648 ) ;
#14989=CARTESIAN_POINT ( 'NONE',  ( -9.403944755730117677, -16.79473832354794993, 16.99999999999999645 ) ) ;
#14990=ORIENTED_EDGE ( 'NONE', *, *, #29, .F. ) ;
#15000=EDGE_LOOP ( 'NONE', ( #12367, #11038, #3973, #2268, #14808, #9896, #13293, #12947, #2040, #5376, #7875, #6902 ) ) ;
#15010=EDGE_CURVE ( 'NONE', #6338, #1813, #1982, .T. ) ;
#15016=EDGE_CURVE ( 'NONE', #11000, #2791, #10965, .T. ) ;
#15019=VERTEX_POINT ( 'NONE', #6666 ) ;
#15039=ORIENTED_EDGE ( 'NONE', *, *, #12553, .F. ) ;
#15045=DIRECTION ( 'NONE',  ( -5.480158469902919838E-17, -1.051478716308701618E-16, -1.000000000000000000 ) ) ;
#15046=LINE ( 'NONE', #4514, #11050 ) ;
#15051=CARTESIAN_POINT ( 'NONE',  ( -9.403944755730119454, -7.794738323547949932, 22.00000000000000000 ) ) ;
#15105=FACE_OUTER_BOUND ( 'NONE', #11009, .T. ) ;
#15127=DIRECTION ( 'NONE',  ( 0.000000000000000000, 1.000000000000000000, -1.084202172485504187E-16 ) ) ;
#15143=CARTESIAN_POINT ( 'NONE',  ( -18.40394475573011945, -10.79473832354794460, -5.000000000000000000 ) ) ;
#15166=CIRCLE ( 'NONE', #11952, 3.799999999999999378 ) ;
#15180=DIRECTION ( 'NONE',  ( -0.6310987668242443727, -0.7757024858236036824, -5.947623346206206400E-19 ) ) ;
#15252=COLOUR_RGB('Light Blue',0.38,0.62,0.78);
#15253=FILL_AREA_STYLE_COLOUR('',#15252);
#15254=FILL_AREA_STYLE('',(#15253));
#15255=SURFACE_STYLE_FILL_AREA(#15254);
#15256=SURFACE_SIDE_STYLE('',(#15255));
#15257=SURFACE_STYLE_USAGE(.BOTH.,#15256);
#15258=PRESENTATION_STYLE_ASSIGNMENT((#15257));
ENDSEC;
END-ISO-10303-21;
